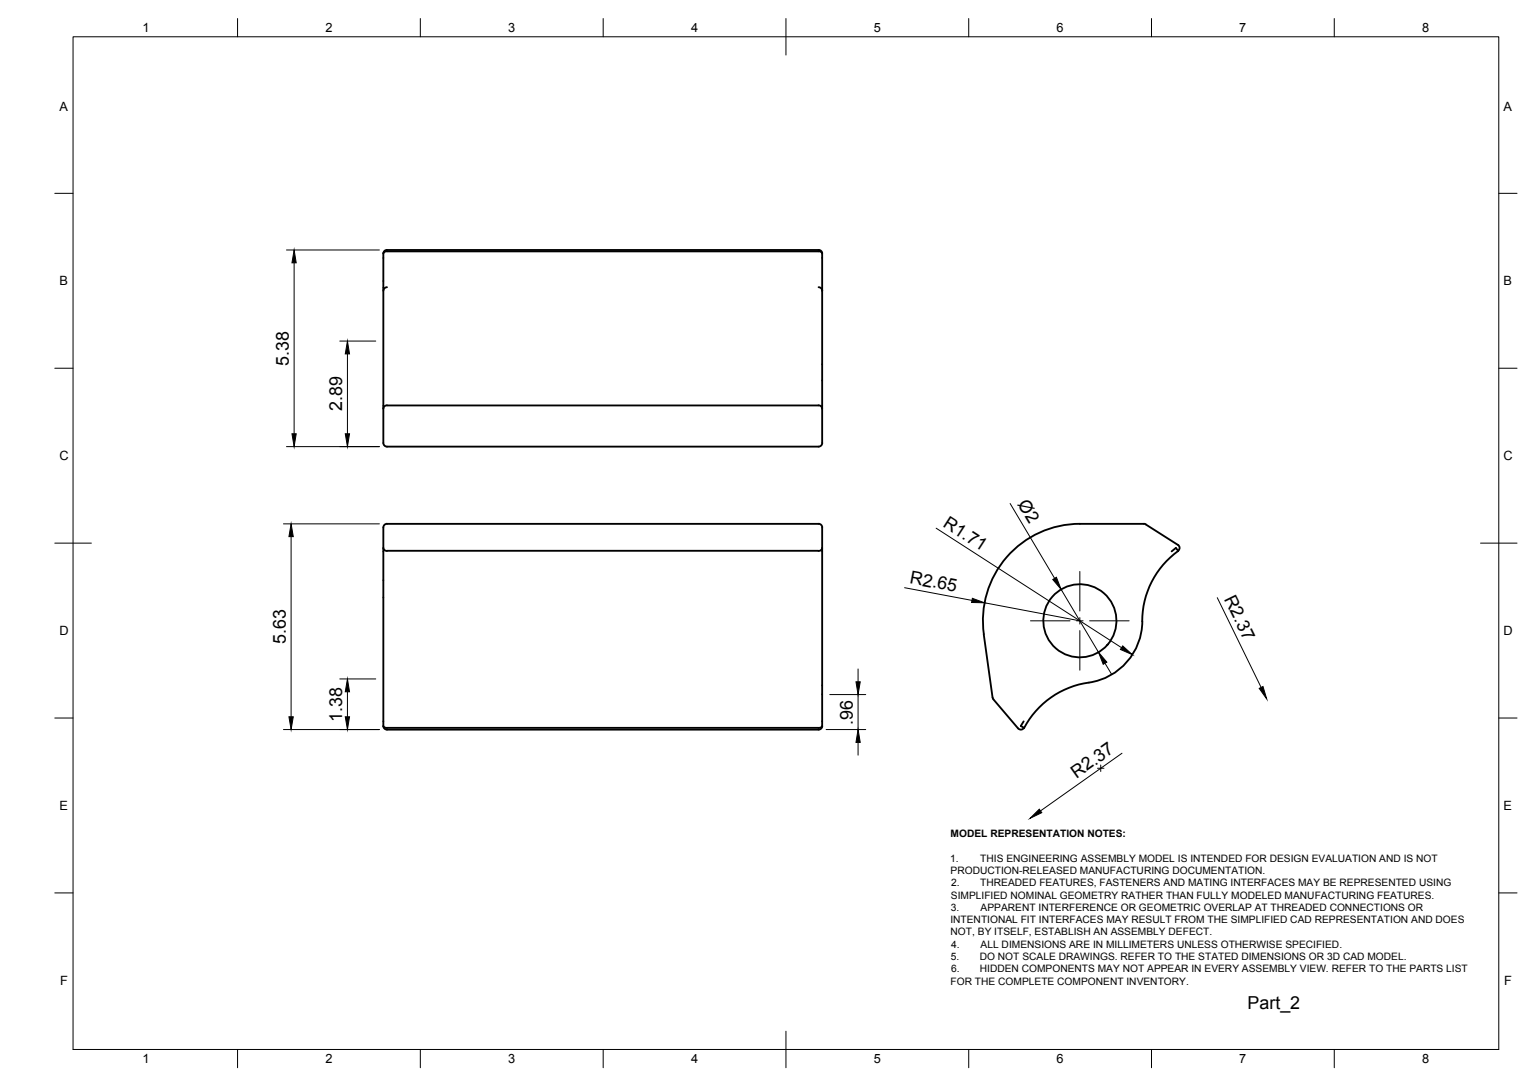
ISO-10303-21;
HEADER;
/* Generated by software containing ST-Developer
 * from STEP Tools, Inc. (www.steptools.com) 
 */

FILE_DESCRIPTION(
/* description */ ('STEP AP242 Edition 2'),
/* implementation_level */ '2;1');

FILE_NAME(
/* name */ 'Part_2.step',
/* time_stamp */ '2026-10-06T10:11:12-07:00',
/* author */ (''),
/* organization */ (''),
/* preprocessor_version */ 'ST-DEVELOPER v20.2',
/* originating_system */ 'Autodesk Translation Framework v15.15.0.0',
/* authorisation */ '');

FILE_SCHEMA (('AUTOMOTIVE_DESIGN { 1 0 10303 214 3 1 1 }'));
ENDSEC;

DATA;
#10=MECHANICAL_DESIGN_GEOMETRIC_PRESENTATION_REPRESENTATION('',(#1798),#54580);
#120=ELLIPSE('',#19218,0.0715418505295819,0.0129149243677278);
#121=ELLIPSE('',#19219,0.0715418505295819,0.0129149243677278);
#122=ELLIPSE('',#19224,0.0715418505290961,0.0129149243676839);
#123=ELLIPSE('',#19225,0.0715418505290961,0.0129149243676839);
#152=SPHERICAL_SURFACE('',#19236,0.0001);
#153=SPHERICAL_SURFACE('',#19238,0.0001);
#154=SPHERICAL_SURFACE('',#19251,0.0001);
#155=SPHERICAL_SURFACE('',#19256,0.0001);
#156=SPHERICAL_SURFACE('',#19270,0.0001);
#157=SPHERICAL_SURFACE('',#19273,0.0001);
#158=SPHERICAL_SURFACE('',#19284,0.0001);
#159=SPHERICAL_SURFACE('',#19286,0.0001);
#273=TOROIDAL_SURFACE('',#19243,0.0024677376190381,9.99991913251056E-5);
#274=TOROIDAL_SURFACE('',#19252,0.00160789487802693,0.0001);
#275=TOROIDAL_SURFACE('',#19254,0.00255162305984738,0.0001);
#276=TOROIDAL_SURFACE('',#19258,0.00246775438595658,9.99991912004813E-5);
#277=TOROIDAL_SURFACE('',#19259,0.00246775438598435,9.99991912004831E-5);
#278=TOROIDAL_SURFACE('',#19268,0.00160789487802693,0.0001);
#279=TOROIDAL_SURFACE('',#19275,0.00255162305984738,0.0001);
#280=TOROIDAL_SURFACE('',#19277,0.00246773761894624,9.99991913251039E-5);
#281=TOROIDAL_SURFACE('',#19289,0.0011,0.0001);
#282=TOROIDAL_SURFACE('',#19291,0.0011,0.0001);
#1352=B_SPLINE_CURVE_WITH_KNOTS('',3,(#48950,#48951,#48952,#48953),
 .UNSPECIFIED.,.F.,.F.,(4,4),(2.77758216759816E-8,0.0598155593219101),
 .UNSPECIFIED.);
#1353=B_SPLINE_CURVE_WITH_KNOTS('',3,(#48955,#48956,#48957,#48958,#48959,
#48960,#48961,#48962,#48963,#48964),.UNSPECIFIED.,.F.,.F.,(4,3,3,4),(0.0598155593219101,
0.400094789280781,0.882156340214427,1.),.UNSPECIFIED.);
#1354=B_SPLINE_CURVE_WITH_KNOTS('',3,(#48989,#48990,#48991,#48992),
 .UNSPECIFIED.,.F.,.F.,(4,4),(2.77758270156303E-8,0.0598155595006793),
 .UNSPECIFIED.);
#1355=B_SPLINE_CURVE_WITH_KNOTS('',3,(#48994,#48995,#48996,#48997,#48998,
#48999,#49000,#49001,#49002,#49003),.UNSPECIFIED.,.F.,.F.,(4,3,3,4),(0.0598155595006793,
0.400094789276241,0.882156340205139,1.),.UNSPECIFIED.);
#1356=B_SPLINE_CURVE_WITH_KNOTS('',3,(#49031,#49032,#49033,#49034,#49035,
#49036,#49037),.UNSPECIFIED.,.F.,.F.,(4,3,4),(0.,0.811097963900528,0.999989357516093),
 .UNSPECIFIED.);
#1357=B_SPLINE_CURVE_WITH_KNOTS('',3,(#49045,#49046,#49047,#49048,#49049,
#49050,#49051),.UNSPECIFIED.,.F.,.F.,(4,3,4),(0.,0.851452914537907,0.999998335389822),
 .UNSPECIFIED.);
#1358=B_SPLINE_CURVE_WITH_KNOTS('',3,(#49060,#49061,#49062,#49063,#49064,
#49065,#49066),.UNSPECIFIED.,.F.,.F.,(4,3,4),(0.000148834785990088,0.811264189000227,
1.),.UNSPECIFIED.);
#1359=B_SPLINE_CURVE_WITH_KNOTS('',3,(#49074,#49075,#49076,#49077,#49078,
#49079,#49080),.UNSPECIFIED.,.F.,.F.,(4,3,4),(1.66717332357201E-6,0.851450337612495,
1.),.UNSPECIFIED.);
#1360=B_SPLINE_CURVE_WITH_KNOTS('',3,(#49082,#49083,#49084,#49085,#49086,
#49087,#49088),.UNSPECIFIED.,.F.,.F.,(4,3,4),(0.00014883478557751,0.81126418904293,
1.),.UNSPECIFIED.);
#1361=B_SPLINE_CURVE_WITH_KNOTS('',3,(#49109,#49110,#49111,#49112,#49113,
#49114,#49115),.UNSPECIFIED.,.F.,.F.,(4,3,4),(0.,0.811097963770035,0.999989357516),
 .UNSPECIFIED.);
#1754=SHAPE_REPRESENTATION_RELATIONSHIP('SRR','None',#54641,#1768);
#1768=ADVANCED_BREP_SHAPE_REPRESENTATION('',(#1812),#54577);
#1798=STYLED_ITEM('',(#54712),#1812);
#1812=MANIFOLD_SOLID_BREP('Body1',#17677);
#2311=LINE('',#48890,#2904);
#2312=LINE('',#48894,#2905);
#2313=LINE('',#48899,#2906);
#2314=LINE('',#48901,#2907);
#2315=LINE('',#48903,#2908);
#2316=LINE('',#48904,#2909);
#2317=LINE('',#48908,#2910);
#2318=LINE('',#48910,#2911);
#2319=LINE('',#48912,#2912);
#2320=LINE('',#48913,#2913);
#2321=LINE('',#48918,#2914);
#2322=LINE('',#48922,#2915);
#2323=LINE('',#48924,#2916);
#2324=LINE('',#48925,#2917);
#2325=LINE('',#48929,#2918);
#2326=LINE('',#48931,#2919);
#2327=LINE('',#48933,#2920);
#2328=LINE('',#48934,#2921);
#2329=LINE('',#48938,#2922);
#2330=LINE('',#48942,#2923);
#2331=LINE('',#48972,#2924);
#2332=LINE('',#48974,#2925);
#2333=LINE('',#48978,#2926);
#2334=LINE('',#48979,#2927);
#2335=LINE('',#48985,#2928);
#2336=LINE('',#48987,#2929);
#2337=LINE('',#49011,#2930);
#2338=LINE('',#49013,#2931);
#2339=LINE('',#49023,#2932);
#2904=VECTOR('',#22829,0.01);
#2905=VECTOR('',#22832,0.01);
#2906=VECTOR('',#22837,1.);
#2907=VECTOR('',#22838,1.);
#2908=VECTOR('',#22839,1.);
#2909=VECTOR('',#22840,1.);
#2910=VECTOR('',#22843,1.);
#2911=VECTOR('',#22844,1.);
#2912=VECTOR('',#22845,1.);
#2913=VECTOR('',#22846,1.);
#2914=VECTOR('',#22851,1.);
#2915=VECTOR('',#22856,1.);
#2916=VECTOR('',#22857,1.);
#2917=VECTOR('',#22858,1.);
#2918=VECTOR('',#22861,1.);
#2919=VECTOR('',#22862,1.);
#2920=VECTOR('',#22863,1.);
#2921=VECTOR('',#22864,1.);
#2922=VECTOR('',#22867,0.01);
#2923=VECTOR('',#22870,0.01);
#2924=VECTOR('',#22887,1.);
#2925=VECTOR('',#22888,1.);
#2926=VECTOR('',#22891,1.);
#2927=VECTOR('',#22892,1.);
#2928=VECTOR('',#22897,1.);
#2929=VECTOR('',#22898,1.);
#2930=VECTOR('',#22905,1.);
#2931=VECTOR('',#22906,1.);
#2932=VECTOR('',#22917,0.001);
#3408=CYLINDRICAL_SURFACE('',#19200,0.00240582032312608);
#3409=CYLINDRICAL_SURFACE('',#19205,0.00265162305984738);
#3410=CYLINDRICAL_SURFACE('',#19210,0.00240582032360216);
#3411=CYLINDRICAL_SURFACE('',#19213,0.00170789487802692);
#3412=CYLINDRICAL_SURFACE('',#19228,0.001);
#3413=CYLINDRICAL_SURFACE('',#19233,0.0001);
#3414=CYLINDRICAL_SURFACE('',#19241,0.0001);
#3415=CYLINDRICAL_SURFACE('',#19244,0.0001);
#3416=CYLINDRICAL_SURFACE('',#19246,0.0001);
#3417=CYLINDRICAL_SURFACE('',#19248,0.0001);
#3418=CYLINDRICAL_SURFACE('',#19260,0.0001);
#3419=CYLINDRICAL_SURFACE('',#19264,0.0001);
#3420=CYLINDRICAL_SURFACE('',#19266,0.0001);
#3421=CYLINDRICAL_SURFACE('',#19278,0.0001);
#3422=CYLINDRICAL_SURFACE('',#19280,0.0001);
#3423=CYLINDRICAL_SURFACE('',#19282,0.0001);
#3424=CYLINDRICAL_SURFACE('',#19288,0.0001);
#3522=FACE_BOUND('',#5409,.T.);
#3523=FACE_BOUND('',#5411,.T.);
#4349=FACE_OUTER_BOUND('',#5400,.T.);
#4350=FACE_OUTER_BOUND('',#5401,.T.);
#4351=FACE_OUTER_BOUND('',#5402,.T.);
#4352=FACE_OUTER_BOUND('',#5403,.T.);
#4353=FACE_OUTER_BOUND('',#5404,.T.);
#4354=FACE_OUTER_BOUND('',#5405,.T.);
#4355=FACE_OUTER_BOUND('',#5406,.T.);
#4356=FACE_OUTER_BOUND('',#5407,.T.);
#4357=FACE_OUTER_BOUND('',#5408,.T.);
#4358=FACE_OUTER_BOUND('',#5410,.T.);
#4359=FACE_OUTER_BOUND('',#5412,.T.);
#4360=FACE_OUTER_BOUND('',#5413,.T.);
#4361=FACE_OUTER_BOUND('',#5414,.T.);
#4362=FACE_OUTER_BOUND('',#5415,.T.);
#4363=FACE_OUTER_BOUND('',#5416,.T.);
#4364=FACE_OUTER_BOUND('',#5417,.T.);
#4365=FACE_OUTER_BOUND('',#5418,.T.);
#4366=FACE_OUTER_BOUND('',#5419,.T.);
#4367=FACE_OUTER_BOUND('',#5420,.T.);
#4368=FACE_OUTER_BOUND('',#5421,.T.);
#4369=FACE_OUTER_BOUND('',#5422,.T.);
#4370=FACE_OUTER_BOUND('',#5423,.T.);
#4371=FACE_OUTER_BOUND('',#5424,.T.);
#4372=FACE_OUTER_BOUND('',#5425,.T.);
#4373=FACE_OUTER_BOUND('',#5426,.T.);
#4374=FACE_OUTER_BOUND('',#5427,.T.);
#4375=FACE_OUTER_BOUND('',#5428,.T.);
#4376=FACE_OUTER_BOUND('',#5429,.T.);
#4377=FACE_OUTER_BOUND('',#5430,.T.);
#4378=FACE_OUTER_BOUND('',#5431,.T.);
#4379=FACE_OUTER_BOUND('',#5432,.T.);
#4380=FACE_OUTER_BOUND('',#5433,.T.);
#4381=FACE_OUTER_BOUND('',#5434,.T.);
#4382=FACE_OUTER_BOUND('',#5435,.T.);
#4383=FACE_OUTER_BOUND('',#5436,.T.);
#4384=FACE_OUTER_BOUND('',#5437,.T.);
#4385=FACE_OUTER_BOUND('',#5438,.T.);
#4386=FACE_OUTER_BOUND('',#5439,.T.);
#4387=FACE_OUTER_BOUND('',#5440,.T.);
#4388=FACE_OUTER_BOUND('',#5441,.T.);
#4389=FACE_OUTER_BOUND('',#5442,.T.);
#5400=EDGE_LOOP('',(#15571,#15572,#15573,#15574));
#5401=EDGE_LOOP('',(#15575,#15576,#15577,#15578));
#5402=EDGE_LOOP('',(#15579,#15580,#15581,#15582));
#5403=EDGE_LOOP('',(#15583,#15584,#15585,#15586));
#5404=EDGE_LOOP('',(#15587,#15588,#15589,#15590));
#5405=EDGE_LOOP('',(#15591,#15592,#15593,#15594));
#5406=EDGE_LOOP('',(#15595,#15596,#15597,#15598));
#5407=EDGE_LOOP('',(#15599,#15600,#15601,#15602));
#5408=EDGE_LOOP('',(#15603,#15604,#15605,#15606,#15607,#15608,#15609,#15610,
#15611,#15612));
#5409=EDGE_LOOP('',(#15613));
#5410=EDGE_LOOP('',(#15614,#15615,#15616,#15617,#15618,#15619,#15620,#15621,
#15622,#15623));
#5411=EDGE_LOOP('',(#15624));
#5412=EDGE_LOOP('',(#15625,#15626,#15627,#15628,#15629,#15630));
#5413=EDGE_LOOP('',(#15631,#15632,#15633,#15634));
#5414=EDGE_LOOP('',(#15635,#15636,#15637));
#5415=EDGE_LOOP('',(#15638,#15639,#15640));
#5416=EDGE_LOOP('',(#15641,#15642,#15643,#15644));
#5417=EDGE_LOOP('',(#15645,#15646,#15647,#15648,#15649));
#5418=EDGE_LOOP('',(#15650,#15651,#15652,#15653));
#5419=EDGE_LOOP('',(#15654,#15655,#15656,#15657));
#5420=EDGE_LOOP('',(#15658,#15659,#15660,#15661));
#5421=EDGE_LOOP('',(#15662,#15663,#15664));
#5422=EDGE_LOOP('',(#15665,#15666,#15667,#15668));
#5423=EDGE_LOOP('',(#15669,#15670,#15671,#15672));
#5424=EDGE_LOOP('',(#15673,#15674,#15675));
#5425=EDGE_LOOP('',(#15676,#15677,#15678,#15679,#15680));
#5426=EDGE_LOOP('',(#15681,#15682,#15683,#15684,#15685));
#5427=EDGE_LOOP('',(#15686,#15687,#15688,#15689,#15690));
#5428=EDGE_LOOP('',(#15691,#15692,#15693,#15694));
#5429=EDGE_LOOP('',(#15695,#15696,#15697,#15698));
#5430=EDGE_LOOP('',(#15699,#15700,#15701,#15702));
#5431=EDGE_LOOP('',(#15703,#15704,#15705,#15706,#15707,#15708));
#5432=EDGE_LOOP('',(#15709,#15710,#15711));
#5433=EDGE_LOOP('',(#15712,#15713,#15714,#15715));
#5434=EDGE_LOOP('',(#15716,#15717,#15718,#15719,#15720));
#5435=EDGE_LOOP('',(#15721,#15722,#15723,#15724));
#5436=EDGE_LOOP('',(#15725,#15726,#15727,#15728));
#5437=EDGE_LOOP('',(#15729,#15730,#15731,#15732));
#5438=EDGE_LOOP('',(#15733,#15734,#15735));
#5439=EDGE_LOOP('',(#15736,#15737,#15738));
#5440=EDGE_LOOP('',(#15739,#15740,#15741,#15742));
#5441=EDGE_LOOP('',(#15743,#15744,#15745,#15746,#15747));
#5442=EDGE_LOOP('',(#15748,#15749,#15750,#15751,#15752));
#6312=CIRCLE('',#19201,0.00236773842762747);
#6313=CIRCLE('',#19202,0.00236775519479021);
#6314=CIRCLE('',#19206,0.00265162305984738);
#6315=CIRCLE('',#19207,0.00265162305984738);
#6316=CIRCLE('',#19211,0.00236775519476243);
#6317=CIRCLE('',#19212,0.00236773842771933);
#6318=CIRCLE('',#19214,0.00170789487802692);
#6319=CIRCLE('',#19215,0.00170789487802692);
#6320=CIRCLE('',#19217,0.00160789487802693);
#6321=CIRCLE('',#19220,0.00255162305984738);
#6322=CIRCLE('',#19221,0.0011);
#6323=CIRCLE('',#19223,0.00160789487802693);
#6324=CIRCLE('',#19226,0.00255162305984738);
#6325=CIRCLE('',#19227,0.0011);
#6326=CIRCLE('',#19229,0.001);
#6327=CIRCLE('',#19230,0.001);
#6328=CIRCLE('',#19231,0.001);
#6329=CIRCLE('',#19232,0.001);
#6330=CIRCLE('',#19234,0.0001);
#6331=CIRCLE('',#19235,0.0001);
#6332=CIRCLE('',#19237,0.0001);
#6333=CIRCLE('',#19239,0.0001);
#6334=CIRCLE('',#19240,0.0001);
#6335=CIRCLE('',#19242,0.0001);
#6336=CIRCLE('',#19245,0.0001);
#6337=CIRCLE('',#19247,0.0001);
#6338=CIRCLE('',#19249,0.0001);
#6339=CIRCLE('',#19250,0.0001);
#6340=CIRCLE('',#19253,0.000100001088290115);
#6341=CIRCLE('',#19255,0.0001);
#6342=CIRCLE('',#19257,0.0001);
#6343=CIRCLE('',#19261,0.0001);
#6344=CIRCLE('',#19262,0.0001);
#6345=CIRCLE('',#19263,0.0001);
#6346=CIRCLE('',#19265,0.0001);
#6347=CIRCLE('',#19267,0.0001);
#6348=CIRCLE('',#19269,0.000100001089498111);
#6349=CIRCLE('',#19271,9.99999999999998E-5);
#6350=CIRCLE('',#19272,0.0001);
#6351=CIRCLE('',#19274,0.0001);
#6352=CIRCLE('',#19276,0.0001);
#6353=CIRCLE('',#19279,0.0001);
#6354=CIRCLE('',#19281,0.0001);
#6355=CIRCLE('',#19283,0.0001);
#6356=CIRCLE('',#19285,0.0001);
#6357=CIRCLE('',#19287,0.0001);
#6358=CIRCLE('',#19290,0.0001);
#6359=CIRCLE('',#19292,0.0001);
#8021=VERTEX_POINT('',#48888);
#8022=VERTEX_POINT('',#48889);
#8023=VERTEX_POINT('',#48891);
#8024=VERTEX_POINT('',#48893);
#8025=VERTEX_POINT('',#48897);
#8026=VERTEX_POINT('',#48898);
#8027=VERTEX_POINT('',#48900);
#8028=VERTEX_POINT('',#48902);
#8029=VERTEX_POINT('',#48906);
#8030=VERTEX_POINT('',#48907);
#8031=VERTEX_POINT('',#48909);
#8032=VERTEX_POINT('',#48911);
#8033=VERTEX_POINT('',#48915);
#8034=VERTEX_POINT('',#48917);
#8035=VERTEX_POINT('',#48921);
#8036=VERTEX_POINT('',#48923);
#8037=VERTEX_POINT('',#48927);
#8038=VERTEX_POINT('',#48928);
#8039=VERTEX_POINT('',#48930);
#8040=VERTEX_POINT('',#48932);
#8041=VERTEX_POINT('',#48936);
#8042=VERTEX_POINT('',#48937);
#8043=VERTEX_POINT('',#48939);
#8044=VERTEX_POINT('',#48941);
#8045=VERTEX_POINT('',#48948);
#8046=VERTEX_POINT('',#48949);
#8047=VERTEX_POINT('',#48954);
#8048=VERTEX_POINT('',#48965);
#8049=VERTEX_POINT('',#48967);
#8050=VERTEX_POINT('',#48969);
#8051=VERTEX_POINT('',#48971);
#8052=VERTEX_POINT('',#48973);
#8053=VERTEX_POINT('',#48975);
#8054=VERTEX_POINT('',#48977);
#8055=VERTEX_POINT('',#48980);
#8056=VERTEX_POINT('',#48983);
#8057=VERTEX_POINT('',#48984);
#8058=VERTEX_POINT('',#48986);
#8059=VERTEX_POINT('',#48988);
#8060=VERTEX_POINT('',#48993);
#8061=VERTEX_POINT('',#49004);
#8062=VERTEX_POINT('',#49006);
#8063=VERTEX_POINT('',#49008);
#8064=VERTEX_POINT('',#49010);
#8065=VERTEX_POINT('',#49012);
#8066=VERTEX_POINT('',#49015);
#8067=VERTEX_POINT('',#49018);
#8068=VERTEX_POINT('',#49019);
#8069=VERTEX_POINT('',#49022);
#8070=VERTEX_POINT('',#49024);
#8071=VERTEX_POINT('',#49091);
#8072=VERTEX_POINT('',#49101);
#10577=EDGE_CURVE('',#8021,#8022,#2311,.T.);
#10578=EDGE_CURVE('',#8022,#8023,#6312,.T.);
#10579=EDGE_CURVE('',#8023,#8024,#2312,.T.);
#10580=EDGE_CURVE('',#8024,#8021,#6313,.T.);
#10581=EDGE_CURVE('',#8025,#8026,#2313,.T.);
#10582=EDGE_CURVE('',#8026,#8027,#2314,.F.);
#10583=EDGE_CURVE('',#8027,#8028,#2315,.F.);
#10584=EDGE_CURVE('',#8028,#8025,#2316,.T.);
#10585=EDGE_CURVE('',#8029,#8030,#2317,.T.);
#10586=EDGE_CURVE('',#8030,#8031,#2318,.T.);
#10587=EDGE_CURVE('',#8032,#8031,#2319,.T.);
#10588=EDGE_CURVE('',#8032,#8029,#2320,.F.);
#10589=EDGE_CURVE('',#8031,#8033,#6314,.F.);
#10590=EDGE_CURVE('',#8034,#8033,#2321,.T.);
#10591=EDGE_CURVE('',#8034,#8032,#6315,.T.);
#10592=EDGE_CURVE('',#8033,#8035,#2322,.T.);
#10593=EDGE_CURVE('',#8035,#8036,#2323,.F.);
#10594=EDGE_CURVE('',#8036,#8034,#2324,.F.);
#10595=EDGE_CURVE('',#8037,#8038,#2325,.F.);
#10596=EDGE_CURVE('',#8038,#8039,#2326,.T.);
#10597=EDGE_CURVE('',#8039,#8040,#2327,.T.);
#10598=EDGE_CURVE('',#8040,#8037,#2328,.F.);
#10599=EDGE_CURVE('',#8041,#8042,#2329,.T.);
#10600=EDGE_CURVE('',#8042,#8043,#6316,.T.);
#10601=EDGE_CURVE('',#8044,#8043,#2330,.F.);
#10602=EDGE_CURVE('',#8044,#8041,#6317,.T.);
#10603=EDGE_CURVE('',#8043,#8022,#6318,.F.);
#10604=EDGE_CURVE('',#8021,#8044,#6319,.T.);
#10605=EDGE_CURVE('',#8045,#8046,#1352,.T.);
#10606=EDGE_CURVE('',#8046,#8047,#1353,.T.);
#10607=EDGE_CURVE('',#8047,#8048,#6320,.F.);
#10608=EDGE_CURVE('',#8048,#8049,#120,.T.);
#10609=EDGE_CURVE('',#8049,#8050,#121,.T.);
#10610=EDGE_CURVE('',#8050,#8051,#2331,.T.);
#10611=EDGE_CURVE('',#8051,#8052,#2332,.T.);
#10612=EDGE_CURVE('',#8052,#8053,#6321,.F.);
#10613=EDGE_CURVE('',#8053,#8054,#2333,.T.);
#10614=EDGE_CURVE('',#8054,#8045,#2334,.T.);
#10615=EDGE_CURVE('',#8055,#8055,#6322,.T.);
#10616=EDGE_CURVE('',#8056,#8057,#2335,.F.);
#10617=EDGE_CURVE('',#8057,#8058,#2336,.F.);
#10618=EDGE_CURVE('',#8058,#8059,#1354,.T.);
#10619=EDGE_CURVE('',#8059,#8060,#1355,.T.);
#10620=EDGE_CURVE('',#8060,#8061,#6323,.T.);
#10621=EDGE_CURVE('',#8061,#8062,#122,.T.);
#10622=EDGE_CURVE('',#8062,#8063,#123,.T.);
#10623=EDGE_CURVE('',#8063,#8064,#2337,.F.);
#10624=EDGE_CURVE('',#8064,#8065,#2338,.F.);
#10625=EDGE_CURVE('',#8065,#8056,#6324,.T.);
#10626=EDGE_CURVE('',#8066,#8066,#6325,.F.);
#10627=EDGE_CURVE('',#8067,#8068,#6326,.T.);
#10628=EDGE_CURVE('',#8068,#8067,#6327,.T.);
#10629=EDGE_CURVE('',#8067,#8069,#2339,.T.);
#10630=EDGE_CURVE('',#8069,#8070,#6328,.F.);
#10631=EDGE_CURVE('',#8070,#8069,#6329,.F.);
#10632=EDGE_CURVE('',#8045,#8037,#6330,.T.);
#10633=EDGE_CURVE('',#8038,#8054,#6331,.T.);
#10634=EDGE_CURVE('',#8045,#8041,#1356,.F.);
#10635=EDGE_CURVE('',#8041,#8037,#6332,.F.);
#10636=EDGE_CURVE('',#8038,#8036,#6333,.F.);
#10637=EDGE_CURVE('',#8036,#8054,#6334,.F.);
#10638=EDGE_CURVE('',#8042,#8040,#6335,.T.);
#10639=EDGE_CURVE('',#8047,#8044,#1357,.F.);
#10640=EDGE_CURVE('',#8034,#8053,#6336,.T.);
#10641=EDGE_CURVE('',#8039,#8035,#6337,.T.);
#10642=EDGE_CURVE('',#8040,#8063,#6338,.T.);
#10643=EDGE_CURVE('',#8064,#8039,#6339,.T.);
#10644=EDGE_CURVE('',#8042,#8063,#1358,.F.);
#10645=EDGE_CURVE('',#8048,#8021,#6340,.F.);
#10646=EDGE_CURVE('',#8032,#8052,#6341,.T.);
#10647=EDGE_CURVE('',#8064,#8035,#6342,.F.);
#10648=EDGE_CURVE('',#8043,#8061,#1359,.F.);
#10649=EDGE_CURVE('',#8050,#8024,#1360,.T.);
#10650=EDGE_CURVE('',#8051,#8027,#6343,.T.);
#10651=EDGE_CURVE('',#8071,#8050,#6344,.T.);
#10652=EDGE_CURVE('',#8028,#8071,#6345,.T.);
#10653=EDGE_CURVE('',#8029,#8051,#6346,.T.);
#10654=EDGE_CURVE('',#8065,#8033,#6347,.T.);
#10655=EDGE_CURVE('',#8022,#8060,#6348,.F.);
#10656=EDGE_CURVE('',#8072,#8071,#6349,.T.);
#10657=EDGE_CURVE('',#8028,#8024,#6350,.F.);
#10658=EDGE_CURVE('',#8029,#8027,#6351,.F.);
#10659=EDGE_CURVE('',#8056,#8031,#6352,.T.);
#10660=EDGE_CURVE('',#8023,#8058,#1361,.T.);
#10661=EDGE_CURVE('',#8025,#8023,#6353,.T.);
#10662=EDGE_CURVE('',#8030,#8026,#6354,.T.);
#10663=EDGE_CURVE('',#8057,#8030,#6355,.T.);
#10664=EDGE_CURVE('',#8025,#8058,#6356,.F.);
#10665=EDGE_CURVE('',#8057,#8026,#6357,.F.);
#10666=EDGE_CURVE('',#8068,#8066,#6358,.T.);
#10667=EDGE_CURVE('',#8055,#8070,#6359,.T.);
#15571=ORIENTED_EDGE('',*,*,#10577,.T.);
#15572=ORIENTED_EDGE('',*,*,#10578,.T.);
#15573=ORIENTED_EDGE('',*,*,#10579,.T.);
#15574=ORIENTED_EDGE('',*,*,#10580,.T.);
#15575=ORIENTED_EDGE('',*,*,#10581,.T.);
#15576=ORIENTED_EDGE('',*,*,#10582,.T.);
#15577=ORIENTED_EDGE('',*,*,#10583,.T.);
#15578=ORIENTED_EDGE('',*,*,#10584,.T.);
#15579=ORIENTED_EDGE('',*,*,#10585,.T.);
#15580=ORIENTED_EDGE('',*,*,#10586,.T.);
#15581=ORIENTED_EDGE('',*,*,#10587,.F.);
#15582=ORIENTED_EDGE('',*,*,#10588,.T.);
#15583=ORIENTED_EDGE('',*,*,#10587,.T.);
#15584=ORIENTED_EDGE('',*,*,#10589,.T.);
#15585=ORIENTED_EDGE('',*,*,#10590,.F.);
#15586=ORIENTED_EDGE('',*,*,#10591,.T.);
#15587=ORIENTED_EDGE('',*,*,#10590,.T.);
#15588=ORIENTED_EDGE('',*,*,#10592,.T.);
#15589=ORIENTED_EDGE('',*,*,#10593,.T.);
#15590=ORIENTED_EDGE('',*,*,#10594,.T.);
#15591=ORIENTED_EDGE('',*,*,#10595,.T.);
#15592=ORIENTED_EDGE('',*,*,#10596,.T.);
#15593=ORIENTED_EDGE('',*,*,#10597,.T.);
#15594=ORIENTED_EDGE('',*,*,#10598,.T.);
#15595=ORIENTED_EDGE('',*,*,#10599,.T.);
#15596=ORIENTED_EDGE('',*,*,#10600,.T.);
#15597=ORIENTED_EDGE('',*,*,#10601,.F.);
#15598=ORIENTED_EDGE('',*,*,#10602,.T.);
#15599=ORIENTED_EDGE('',*,*,#10601,.T.);
#15600=ORIENTED_EDGE('',*,*,#10603,.T.);
#15601=ORIENTED_EDGE('',*,*,#10577,.F.);
#15602=ORIENTED_EDGE('',*,*,#10604,.T.);
#15603=ORIENTED_EDGE('',*,*,#10605,.T.);
#15604=ORIENTED_EDGE('',*,*,#10606,.T.);
#15605=ORIENTED_EDGE('',*,*,#10607,.T.);
#15606=ORIENTED_EDGE('',*,*,#10608,.T.);
#15607=ORIENTED_EDGE('',*,*,#10609,.T.);
#15608=ORIENTED_EDGE('',*,*,#10610,.T.);
#15609=ORIENTED_EDGE('',*,*,#10611,.T.);
#15610=ORIENTED_EDGE('',*,*,#10612,.T.);
#15611=ORIENTED_EDGE('',*,*,#10613,.T.);
#15612=ORIENTED_EDGE('',*,*,#10614,.T.);
#15613=ORIENTED_EDGE('',*,*,#10615,.T.);
#15614=ORIENTED_EDGE('',*,*,#10616,.T.);
#15615=ORIENTED_EDGE('',*,*,#10617,.T.);
#15616=ORIENTED_EDGE('',*,*,#10618,.T.);
#15617=ORIENTED_EDGE('',*,*,#10619,.T.);
#15618=ORIENTED_EDGE('',*,*,#10620,.T.);
#15619=ORIENTED_EDGE('',*,*,#10621,.T.);
#15620=ORIENTED_EDGE('',*,*,#10622,.T.);
#15621=ORIENTED_EDGE('',*,*,#10623,.T.);
#15622=ORIENTED_EDGE('',*,*,#10624,.T.);
#15623=ORIENTED_EDGE('',*,*,#10625,.T.);
#15624=ORIENTED_EDGE('',*,*,#10626,.T.);
#15625=ORIENTED_EDGE('',*,*,#10627,.T.);
#15626=ORIENTED_EDGE('',*,*,#10628,.T.);
#15627=ORIENTED_EDGE('',*,*,#10629,.T.);
#15628=ORIENTED_EDGE('',*,*,#10630,.T.);
#15629=ORIENTED_EDGE('',*,*,#10631,.T.);
#15630=ORIENTED_EDGE('',*,*,#10629,.F.);
#15631=ORIENTED_EDGE('',*,*,#10632,.F.);
#15632=ORIENTED_EDGE('',*,*,#10614,.F.);
#15633=ORIENTED_EDGE('',*,*,#10633,.F.);
#15634=ORIENTED_EDGE('',*,*,#10595,.F.);
#15635=ORIENTED_EDGE('',*,*,#10634,.F.);
#15636=ORIENTED_EDGE('',*,*,#10632,.T.);
#15637=ORIENTED_EDGE('',*,*,#10635,.F.);
#15638=ORIENTED_EDGE('',*,*,#10636,.F.);
#15639=ORIENTED_EDGE('',*,*,#10633,.T.);
#15640=ORIENTED_EDGE('',*,*,#10637,.F.);
#15641=ORIENTED_EDGE('',*,*,#10635,.T.);
#15642=ORIENTED_EDGE('',*,*,#10598,.F.);
#15643=ORIENTED_EDGE('',*,*,#10638,.F.);
#15644=ORIENTED_EDGE('',*,*,#10599,.F.);
#15645=ORIENTED_EDGE('',*,*,#10634,.T.);
#15646=ORIENTED_EDGE('',*,*,#10602,.F.);
#15647=ORIENTED_EDGE('',*,*,#10639,.F.);
#15648=ORIENTED_EDGE('',*,*,#10606,.F.);
#15649=ORIENTED_EDGE('',*,*,#10605,.F.);
#15650=ORIENTED_EDGE('',*,*,#10637,.T.);
#15651=ORIENTED_EDGE('',*,*,#10613,.F.);
#15652=ORIENTED_EDGE('',*,*,#10640,.F.);
#15653=ORIENTED_EDGE('',*,*,#10594,.F.);
#15654=ORIENTED_EDGE('',*,*,#10636,.T.);
#15655=ORIENTED_EDGE('',*,*,#10593,.F.);
#15656=ORIENTED_EDGE('',*,*,#10641,.F.);
#15657=ORIENTED_EDGE('',*,*,#10596,.F.);
#15658=ORIENTED_EDGE('',*,*,#10642,.F.);
#15659=ORIENTED_EDGE('',*,*,#10597,.F.);
#15660=ORIENTED_EDGE('',*,*,#10643,.F.);
#15661=ORIENTED_EDGE('',*,*,#10623,.F.);
#15662=ORIENTED_EDGE('',*,*,#10638,.T.);
#15663=ORIENTED_EDGE('',*,*,#10642,.T.);
#15664=ORIENTED_EDGE('',*,*,#10644,.F.);
#15665=ORIENTED_EDGE('',*,*,#10639,.T.);
#15666=ORIENTED_EDGE('',*,*,#10604,.F.);
#15667=ORIENTED_EDGE('',*,*,#10645,.F.);
#15668=ORIENTED_EDGE('',*,*,#10607,.F.);
#15669=ORIENTED_EDGE('',*,*,#10640,.T.);
#15670=ORIENTED_EDGE('',*,*,#10612,.F.);
#15671=ORIENTED_EDGE('',*,*,#10646,.F.);
#15672=ORIENTED_EDGE('',*,*,#10591,.F.);
#15673=ORIENTED_EDGE('',*,*,#10643,.T.);
#15674=ORIENTED_EDGE('',*,*,#10641,.T.);
#15675=ORIENTED_EDGE('',*,*,#10647,.F.);
#15676=ORIENTED_EDGE('',*,*,#10644,.T.);
#15677=ORIENTED_EDGE('',*,*,#10622,.F.);
#15678=ORIENTED_EDGE('',*,*,#10621,.F.);
#15679=ORIENTED_EDGE('',*,*,#10648,.F.);
#15680=ORIENTED_EDGE('',*,*,#10600,.F.);
#15681=ORIENTED_EDGE('',*,*,#10645,.T.);
#15682=ORIENTED_EDGE('',*,*,#10580,.F.);
#15683=ORIENTED_EDGE('',*,*,#10649,.F.);
#15684=ORIENTED_EDGE('',*,*,#10609,.F.);
#15685=ORIENTED_EDGE('',*,*,#10608,.F.);
#15686=ORIENTED_EDGE('',*,*,#10650,.F.);
#15687=ORIENTED_EDGE('',*,*,#10610,.F.);
#15688=ORIENTED_EDGE('',*,*,#10651,.F.);
#15689=ORIENTED_EDGE('',*,*,#10652,.F.);
#15690=ORIENTED_EDGE('',*,*,#10583,.F.);
#15691=ORIENTED_EDGE('',*,*,#10646,.T.);
#15692=ORIENTED_EDGE('',*,*,#10611,.F.);
#15693=ORIENTED_EDGE('',*,*,#10653,.F.);
#15694=ORIENTED_EDGE('',*,*,#10588,.F.);
#15695=ORIENTED_EDGE('',*,*,#10647,.T.);
#15696=ORIENTED_EDGE('',*,*,#10592,.F.);
#15697=ORIENTED_EDGE('',*,*,#10654,.F.);
#15698=ORIENTED_EDGE('',*,*,#10624,.F.);
#15699=ORIENTED_EDGE('',*,*,#10648,.T.);
#15700=ORIENTED_EDGE('',*,*,#10620,.F.);
#15701=ORIENTED_EDGE('',*,*,#10655,.F.);
#15702=ORIENTED_EDGE('',*,*,#10603,.F.);
#15703=ORIENTED_EDGE('',*,*,#10652,.T.);
#15704=ORIENTED_EDGE('',*,*,#10656,.F.);
#15705=ORIENTED_EDGE('',*,*,#10656,.T.);
#15706=ORIENTED_EDGE('',*,*,#10651,.T.);
#15707=ORIENTED_EDGE('',*,*,#10649,.T.);
#15708=ORIENTED_EDGE('',*,*,#10657,.F.);
#15709=ORIENTED_EDGE('',*,*,#10653,.T.);
#15710=ORIENTED_EDGE('',*,*,#10650,.T.);
#15711=ORIENTED_EDGE('',*,*,#10658,.F.);
#15712=ORIENTED_EDGE('',*,*,#10654,.T.);
#15713=ORIENTED_EDGE('',*,*,#10589,.F.);
#15714=ORIENTED_EDGE('',*,*,#10659,.F.);
#15715=ORIENTED_EDGE('',*,*,#10625,.F.);
#15716=ORIENTED_EDGE('',*,*,#10655,.T.);
#15717=ORIENTED_EDGE('',*,*,#10619,.F.);
#15718=ORIENTED_EDGE('',*,*,#10618,.F.);
#15719=ORIENTED_EDGE('',*,*,#10660,.F.);
#15720=ORIENTED_EDGE('',*,*,#10578,.F.);
#15721=ORIENTED_EDGE('',*,*,#10657,.T.);
#15722=ORIENTED_EDGE('',*,*,#10579,.F.);
#15723=ORIENTED_EDGE('',*,*,#10661,.F.);
#15724=ORIENTED_EDGE('',*,*,#10584,.F.);
#15725=ORIENTED_EDGE('',*,*,#10658,.T.);
#15726=ORIENTED_EDGE('',*,*,#10582,.F.);
#15727=ORIENTED_EDGE('',*,*,#10662,.F.);
#15728=ORIENTED_EDGE('',*,*,#10585,.F.);
#15729=ORIENTED_EDGE('',*,*,#10659,.T.);
#15730=ORIENTED_EDGE('',*,*,#10586,.F.);
#15731=ORIENTED_EDGE('',*,*,#10663,.F.);
#15732=ORIENTED_EDGE('',*,*,#10616,.F.);
#15733=ORIENTED_EDGE('',*,*,#10661,.T.);
#15734=ORIENTED_EDGE('',*,*,#10660,.T.);
#15735=ORIENTED_EDGE('',*,*,#10664,.F.);
#15736=ORIENTED_EDGE('',*,*,#10663,.T.);
#15737=ORIENTED_EDGE('',*,*,#10662,.T.);
#15738=ORIENTED_EDGE('',*,*,#10665,.F.);
#15739=ORIENTED_EDGE('',*,*,#10664,.T.);
#15740=ORIENTED_EDGE('',*,*,#10617,.F.);
#15741=ORIENTED_EDGE('',*,*,#10665,.T.);
#15742=ORIENTED_EDGE('',*,*,#10581,.F.);
#15743=ORIENTED_EDGE('',*,*,#10627,.F.);
#15744=ORIENTED_EDGE('',*,*,#10628,.F.);
#15745=ORIENTED_EDGE('',*,*,#10666,.T.);
#15746=ORIENTED_EDGE('',*,*,#10626,.F.);
#15747=ORIENTED_EDGE('',*,*,#10666,.F.);
#15748=ORIENTED_EDGE('',*,*,#10615,.F.);
#15749=ORIENTED_EDGE('',*,*,#10667,.T.);
#15750=ORIENTED_EDGE('',*,*,#10630,.F.);
#15751=ORIENTED_EDGE('',*,*,#10631,.F.);
#15752=ORIENTED_EDGE('',*,*,#10667,.F.);
#16639=PLANE('',#19203);
#16640=PLANE('',#19204);
#16641=PLANE('',#19208);
#16642=PLANE('',#19209);
#16643=PLANE('',#19216);
#16644=PLANE('',#19222);
#17465=ADVANCED_FACE('',(#4349),#3408,.F.);
#17466=ADVANCED_FACE('',(#4350),#16639,.F.);
#17467=ADVANCED_FACE('',(#4351),#16640,.F.);
#17468=ADVANCED_FACE('',(#4352),#3409,.T.);
#17469=ADVANCED_FACE('',(#4353),#16641,.F.);
#17470=ADVANCED_FACE('',(#4354),#16642,.F.);
#17471=ADVANCED_FACE('',(#4355),#3410,.F.);
#17472=ADVANCED_FACE('',(#4356),#3411,.T.);
#17473=ADVANCED_FACE('',(#4357,#3522),#16643,.F.);
#17474=ADVANCED_FACE('',(#4358,#3523),#16644,.T.);
#17475=ADVANCED_FACE('',(#4359),#3412,.F.);
#17476=ADVANCED_FACE('',(#4360),#3413,.T.);
#17477=ADVANCED_FACE('',(#4361),#152,.T.);
#17478=ADVANCED_FACE('',(#4362),#153,.T.);
#17479=ADVANCED_FACE('',(#4363),#3414,.T.);
#17480=ADVANCED_FACE('',(#4364),#273,.T.);
#17481=ADVANCED_FACE('',(#4365),#3415,.T.);
#17482=ADVANCED_FACE('',(#4366),#3416,.T.);
#17483=ADVANCED_FACE('',(#4367),#3417,.T.);
#17484=ADVANCED_FACE('',(#4368),#154,.T.);
#17485=ADVANCED_FACE('',(#4369),#274,.T.);
#17486=ADVANCED_FACE('',(#4370),#275,.T.);
#17487=ADVANCED_FACE('',(#4371),#155,.T.);
#17488=ADVANCED_FACE('',(#4372),#276,.T.);
#17489=ADVANCED_FACE('',(#4373),#277,.T.);
#17490=ADVANCED_FACE('',(#4374),#3418,.T.);
#17491=ADVANCED_FACE('',(#4375),#3419,.T.);
#17492=ADVANCED_FACE('',(#4376),#3420,.T.);
#17493=ADVANCED_FACE('',(#4377),#278,.T.);
#17494=ADVANCED_FACE('',(#4378),#156,.T.);
#17495=ADVANCED_FACE('',(#4379),#157,.T.);
#17496=ADVANCED_FACE('',(#4380),#279,.T.);
#17497=ADVANCED_FACE('',(#4381),#280,.T.);
#17498=ADVANCED_FACE('',(#4382),#3421,.T.);
#17499=ADVANCED_FACE('',(#4383),#3422,.T.);
#17500=ADVANCED_FACE('',(#4384),#3423,.T.);
#17501=ADVANCED_FACE('',(#4385),#158,.T.);
#17502=ADVANCED_FACE('',(#4386),#159,.T.);
#17503=ADVANCED_FACE('',(#4387),#3424,.T.);
#17504=ADVANCED_FACE('',(#4388),#281,.T.);
#17505=ADVANCED_FACE('',(#4389),#282,.T.);
#17677=CLOSED_SHELL('',(#17465,#17466,#17467,#17468,#17469,#17470,#17471,
#17472,#17473,#17474,#17475,#17476,#17477,#17478,#17479,#17480,#17481,#17482,
#17483,#17484,#17485,#17486,#17487,#17488,#17489,#17490,#17491,#17492,#17493,
#17494,#17495,#17496,#17497,#17498,#17499,#17500,#17501,#17502,#17503,#17504,
#17505));
#19199=AXIS2_PLACEMENT_3D('',#48886,#22825,#22826);
#19200=AXIS2_PLACEMENT_3D('',#48887,#22827,#22828);
#19201=AXIS2_PLACEMENT_3D('',#48892,#22830,#22831);
#19202=AXIS2_PLACEMENT_3D('',#48895,#22833,#22834);
#19203=AXIS2_PLACEMENT_3D('',#48896,#22835,#22836);
#19204=AXIS2_PLACEMENT_3D('',#48905,#22841,#22842);
#19205=AXIS2_PLACEMENT_3D('',#48914,#22847,#22848);
#19206=AXIS2_PLACEMENT_3D('',#48916,#22849,#22850);
#19207=AXIS2_PLACEMENT_3D('',#48919,#22852,#22853);
#19208=AXIS2_PLACEMENT_3D('',#48920,#22854,#22855);
#19209=AXIS2_PLACEMENT_3D('',#48926,#22859,#22860);
#19210=AXIS2_PLACEMENT_3D('',#48935,#22865,#22866);
#19211=AXIS2_PLACEMENT_3D('',#48940,#22868,#22869);
#19212=AXIS2_PLACEMENT_3D('',#48943,#22871,#22872);
#19213=AXIS2_PLACEMENT_3D('',#48944,#22873,#22874);
#19214=AXIS2_PLACEMENT_3D('',#48945,#22875,#22876);
#19215=AXIS2_PLACEMENT_3D('',#48946,#22877,#22878);
#19216=AXIS2_PLACEMENT_3D('',#48947,#22879,#22880);
#19217=AXIS2_PLACEMENT_3D('',#48966,#22881,#22882);
#19218=AXIS2_PLACEMENT_3D('',#48968,#22883,#22884);
#19219=AXIS2_PLACEMENT_3D('',#48970,#22885,#22886);
#19220=AXIS2_PLACEMENT_3D('',#48976,#22889,#22890);
#19221=AXIS2_PLACEMENT_3D('',#48981,#22893,#22894);
#19222=AXIS2_PLACEMENT_3D('',#48982,#22895,#22896);
#19223=AXIS2_PLACEMENT_3D('',#49005,#22899,#22900);
#19224=AXIS2_PLACEMENT_3D('',#49007,#22901,#22902);
#19225=AXIS2_PLACEMENT_3D('',#49009,#22903,#22904);
#19226=AXIS2_PLACEMENT_3D('',#49014,#22907,#22908);
#19227=AXIS2_PLACEMENT_3D('',#49016,#22909,#22910);
#19228=AXIS2_PLACEMENT_3D('',#49017,#22911,#22912);
#19229=AXIS2_PLACEMENT_3D('',#49020,#22913,#22914);
#19230=AXIS2_PLACEMENT_3D('',#49021,#22915,#22916);
#19231=AXIS2_PLACEMENT_3D('',#49025,#22918,#22919);
#19232=AXIS2_PLACEMENT_3D('',#49026,#22920,#22921);
#19233=AXIS2_PLACEMENT_3D('',#49027,#22922,#22923);
#19234=AXIS2_PLACEMENT_3D('',#49028,#22924,#22925);
#19235=AXIS2_PLACEMENT_3D('',#49029,#22926,#22927);
#19236=AXIS2_PLACEMENT_3D('',#49030,#22928,#22929);
#19237=AXIS2_PLACEMENT_3D('',#49038,#22930,#22931);
#19238=AXIS2_PLACEMENT_3D('',#49039,#22932,#22933);
#19239=AXIS2_PLACEMENT_3D('',#49040,#22934,#22935);
#19240=AXIS2_PLACEMENT_3D('',#49041,#22936,#22937);
#19241=AXIS2_PLACEMENT_3D('',#49042,#22938,#22939);
#19242=AXIS2_PLACEMENT_3D('',#49043,#22940,#22941);
#19243=AXIS2_PLACEMENT_3D('',#49044,#22942,#22943);
#19244=AXIS2_PLACEMENT_3D('',#49052,#22944,#22945);
#19245=AXIS2_PLACEMENT_3D('',#49053,#22946,#22947);
#19246=AXIS2_PLACEMENT_3D('',#49054,#22948,#22949);
#19247=AXIS2_PLACEMENT_3D('',#49055,#22950,#22951);
#19248=AXIS2_PLACEMENT_3D('',#49056,#22952,#22953);
#19249=AXIS2_PLACEMENT_3D('',#49057,#22954,#22955);
#19250=AXIS2_PLACEMENT_3D('',#49058,#22956,#22957);
#19251=AXIS2_PLACEMENT_3D('',#49059,#22958,#22959);
#19252=AXIS2_PLACEMENT_3D('',#49067,#22960,#22961);
#19253=AXIS2_PLACEMENT_3D('',#49068,#22962,#22963);
#19254=AXIS2_PLACEMENT_3D('',#49069,#22964,#22965);
#19255=AXIS2_PLACEMENT_3D('',#49070,#22966,#22967);
#19256=AXIS2_PLACEMENT_3D('',#49071,#22968,#22969);
#19257=AXIS2_PLACEMENT_3D('',#49072,#22970,#22971);
#19258=AXIS2_PLACEMENT_3D('',#49073,#22972,#22973);
#19259=AXIS2_PLACEMENT_3D('',#49081,#22974,#22975);
#19260=AXIS2_PLACEMENT_3D('',#49089,#22976,#22977);
#19261=AXIS2_PLACEMENT_3D('',#49090,#22978,#22979);
#19262=AXIS2_PLACEMENT_3D('',#49092,#22980,#22981);
#19263=AXIS2_PLACEMENT_3D('',#49093,#22982,#22983);
#19264=AXIS2_PLACEMENT_3D('',#49094,#22984,#22985);
#19265=AXIS2_PLACEMENT_3D('',#49095,#22986,#22987);
#19266=AXIS2_PLACEMENT_3D('',#49096,#22988,#22989);
#19267=AXIS2_PLACEMENT_3D('',#49097,#22990,#22991);
#19268=AXIS2_PLACEMENT_3D('',#49098,#22992,#22993);
#19269=AXIS2_PLACEMENT_3D('',#49099,#22994,#22995);
#19270=AXIS2_PLACEMENT_3D('',#49100,#22996,#22997);
#19271=AXIS2_PLACEMENT_3D('',#49102,#22998,#22999);
#19272=AXIS2_PLACEMENT_3D('',#49103,#23000,#23001);
#19273=AXIS2_PLACEMENT_3D('',#49104,#23002,#23003);
#19274=AXIS2_PLACEMENT_3D('',#49105,#23004,#23005);
#19275=AXIS2_PLACEMENT_3D('',#49106,#23006,#23007);
#19276=AXIS2_PLACEMENT_3D('',#49107,#23008,#23009);
#19277=AXIS2_PLACEMENT_3D('',#49108,#23010,#23011);
#19278=AXIS2_PLACEMENT_3D('',#49116,#23012,#23013);
#19279=AXIS2_PLACEMENT_3D('',#49117,#23014,#23015);
#19280=AXIS2_PLACEMENT_3D('',#49118,#23016,#23017);
#19281=AXIS2_PLACEMENT_3D('',#49119,#23018,#23019);
#19282=AXIS2_PLACEMENT_3D('',#49120,#23020,#23021);
#19283=AXIS2_PLACEMENT_3D('',#49121,#23022,#23023);
#19284=AXIS2_PLACEMENT_3D('',#49122,#23024,#23025);
#19285=AXIS2_PLACEMENT_3D('',#49123,#23026,#23027);
#19286=AXIS2_PLACEMENT_3D('',#49124,#23028,#23029);
#19287=AXIS2_PLACEMENT_3D('',#49125,#23030,#23031);
#19288=AXIS2_PLACEMENT_3D('',#49126,#23032,#23033);
#19289=AXIS2_PLACEMENT_3D('',#49127,#23034,#23035);
#19290=AXIS2_PLACEMENT_3D('',#49128,#23036,#23037);
#19291=AXIS2_PLACEMENT_3D('',#49129,#23038,#23039);
#19292=AXIS2_PLACEMENT_3D('',#49130,#23040,#23041);
#22825=DIRECTION('axis',(0.,0.,1.));
#22826=DIRECTION('refdir',(1.,0.,0.));
#22827=DIRECTION('center_axis',(1.24100495794237E-20,1.,9.9579925010296E-17));
#22828=DIRECTION('ref_axis',(-0.242093751695761,9.66207115918887E-17,-0.970252861572627));
#22829=DIRECTION('',(0.,-1.,0.));
#22830=DIRECTION('center_axis',(4.78776181462468E-8,-0.999999999999989,
1.38777575295897E-7));
#22831=DIRECTION('ref_axis',(0.228625617239181,-1.2415592080664E-7,-0.973514420613268));
#22832=DIRECTION('',(0.,1.,0.));
#22833=DIRECTION('center_axis',(4.78638686561428E-8,0.999999999999989,1.38744664442357E-7));
#22834=DIRECTION('ref_axis',(-0.657176856530054,1.36031932324909E-7,-0.753736412309541));
#22835=DIRECTION('center_axis',(-0.988756381047007,0.,0.149535343443703));
#22836=DIRECTION('ref_axis',(0.149535343443703,0.,0.988756381047007));
#22837=DIRECTION('',(-0.149535343443703,0.,-0.988756381047007));
#22838=DIRECTION('',(0.,-1.,0.));
#22839=DIRECTION('',(-0.149535343443703,0.,-0.988756381047007));
#22840=DIRECTION('',(0.,-1.,0.));
#22841=DIRECTION('center_axis',(-0.754320837054538,0.,0.656505959443889));
#22842=DIRECTION('ref_axis',(0.656505959443889,0.,0.754320837054538));
#22843=DIRECTION('',(0.,-1.,0.));
#22844=DIRECTION('',(-0.656505959443889,0.,-0.754320837054538));
#22845=DIRECTION('',(0.,-1.,0.));
#22846=DIRECTION('',(-0.656505959443889,0.,-0.754320837054538));
#22847=DIRECTION('center_axis',(0.,-1.,0.));
#22848=DIRECTION('ref_axis',(0.,0.,-1.));
#22849=DIRECTION('center_axis',(0.,-1.,0.));
#22850=DIRECTION('ref_axis',(0.,0.,-1.));
#22851=DIRECTION('',(0.,-1.,0.));
#22852=DIRECTION('center_axis',(0.,-1.,0.));
#22853=DIRECTION('ref_axis',(0.,0.,-1.));
#22854=DIRECTION('center_axis',(0.754320837054538,0.,0.656505959443889));
#22855=DIRECTION('ref_axis',(0.656505959443889,0.,-0.754320837054538));
#22856=DIRECTION('',(-0.656505959443889,0.,0.754320837054538));
#22857=DIRECTION('',(0.,-1.,0.));
#22858=DIRECTION('',(-0.656505959443889,0.,0.754320837054538));
#22859=DIRECTION('center_axis',(0.988756381047007,0.,0.149535343443703));
#22860=DIRECTION('ref_axis',(0.149535343443703,0.,-0.988756381047007));
#22861=DIRECTION('',(-0.149535343443703,0.,0.988756381047007));
#22862=DIRECTION('',(0.,-1.,0.));
#22863=DIRECTION('',(-0.149535343443703,0.,0.988756381047007));
#22864=DIRECTION('',(0.,-1.,0.));
#22865=DIRECTION('center_axis',(-1.24149291915094E-20,1.,9.9579925010296E-17));
#22866=DIRECTION('ref_axis',(0.242093751716637,9.66207127726939E-17,-0.970252861567418));
#22867=DIRECTION('',(0.,-1.,0.));
#22868=DIRECTION('center_axis',(-4.78638689058599E-8,-0.999999999999989,
1.38744669549957E-7));
#22869=DIRECTION('ref_axis',(0.657176856532881,-1.36031936363378E-7,-0.753736412307076));
#22870=DIRECTION('',(0.,1.,0.));
#22871=DIRECTION('center_axis',(-4.78776226059778E-8,0.999999999999989,
1.38777586767972E-7));
#22872=DIRECTION('ref_axis',(-0.228625617218267,1.24155931198126E-7,-0.97351442061818));
#22873=DIRECTION('center_axis',(0.,-1.,0.));
#22874=DIRECTION('ref_axis',(-4.27550288255207E-14,0.,1.));
#22875=DIRECTION('center_axis',(0.,-1.,0.));
#22876=DIRECTION('ref_axis',(0.,0.,-1.));
#22877=DIRECTION('center_axis',(0.,-1.,0.));
#22878=DIRECTION('ref_axis',(0.,0.,-1.));
#22879=DIRECTION('center_axis',(0.,-1.,0.));
#22880=DIRECTION('ref_axis',(0.,0.,-1.));
#22881=DIRECTION('center_axis',(0.,-1.,0.));
#22882=DIRECTION('ref_axis',(0.,0.,-1.));
#22883=DIRECTION('center_axis',(0.,-1.,0.));
#22884=DIRECTION('ref_axis',(-0.319023595909223,0.,-0.947746772747419));
#22885=DIRECTION('center_axis',(0.,-1.,0.));
#22886=DIRECTION('ref_axis',(-0.319023595909223,0.,-0.947746772747419));
#22887=DIRECTION('',(-0.149535343443703,0.,-0.988756381047007));
#22888=DIRECTION('',(-0.656505959443889,0.,-0.754320837054538));
#22889=DIRECTION('center_axis',(0.,-1.,0.));
#22890=DIRECTION('ref_axis',(0.,0.,-1.));
#22891=DIRECTION('',(-0.656505959443889,0.,0.754320837054538));
#22892=DIRECTION('',(-0.149535343443703,0.,0.988756381047007));
#22893=DIRECTION('center_axis',(0.,-1.,0.));
#22894=DIRECTION('ref_axis',(0.,0.,-1.));
#22895=DIRECTION('center_axis',(0.,-1.,0.));
#22896=DIRECTION('ref_axis',(0.,0.,-1.));
#22897=DIRECTION('',(-0.656505959443889,0.,-0.754320837054538));
#22898=DIRECTION('',(-0.149535343443703,0.,-0.988756381047007));
#22899=DIRECTION('center_axis',(0.,-1.,0.));
#22900=DIRECTION('ref_axis',(0.,0.,-1.));
#22901=DIRECTION('center_axis',(0.,1.,0.));
#22902=DIRECTION('ref_axis',(-0.319023595909249,0.,0.94774677274741));
#22903=DIRECTION('center_axis',(0.,1.,0.));
#22904=DIRECTION('ref_axis',(-0.319023595909249,0.,0.94774677274741));
#22905=DIRECTION('',(-0.149535343443703,0.,0.988756381047007));
#22906=DIRECTION('',(-0.656505959443889,0.,0.754320837054538));
#22907=DIRECTION('center_axis',(0.,-1.,0.));
#22908=DIRECTION('ref_axis',(0.,0.,-1.));
#22909=DIRECTION('center_axis',(0.,-1.,0.));
#22910=DIRECTION('ref_axis',(0.,0.,-1.));
#22911=DIRECTION('center_axis',(0.,1.,0.));
#22912=DIRECTION('ref_axis',(0.,0.,1.));
#22913=DIRECTION('center_axis',(0.,-1.,0.));
#22914=DIRECTION('ref_axis',(0.,0.,-1.));
#22915=DIRECTION('center_axis',(0.,-1.,0.));
#22916=DIRECTION('ref_axis',(0.,0.,-1.));
#22917=DIRECTION('',(0.,1.,0.));
#22918=DIRECTION('center_axis',(0.,-1.,0.));
#22919=DIRECTION('ref_axis',(0.,0.,-1.));
#22920=DIRECTION('center_axis',(0.,-1.,0.));
#22921=DIRECTION('ref_axis',(0.,0.,-1.));
#22922=DIRECTION('center_axis',(-0.149535343443703,0.,0.988756381047007));
#22923=DIRECTION('ref_axis',(0.988756381047007,0.,0.149535343443703));
#22924=DIRECTION('center_axis',(-0.149535343443704,0.,0.988756381047007));
#22925=DIRECTION('ref_axis',(0.988756381047007,0.,0.149535343443704));
#22926=DIRECTION('center_axis',(0.149535343443704,5.36005908195038E-16,
-0.988756381047007));
#22927=DIRECTION('ref_axis',(-0.988756381047007,1.21230624919584E-32,-0.149535343443704));
#22928=DIRECTION('center_axis',(0.577350269189623,0.577350269189631,0.577350269189624));
#22929=DIRECTION('ref_axis',(-0.707106781186548,0.,0.707106781186547));
#22930=DIRECTION('center_axis',(0.,1.,0.));
#22931=DIRECTION('ref_axis',(0.,0.,1.));
#22932=DIRECTION('center_axis',(0.,1.,0.));
#22933=DIRECTION('ref_axis',(0.,0.,1.));
#22934=DIRECTION('center_axis',(0.,1.,0.));
#22935=DIRECTION('ref_axis',(0.,0.,1.));
#22936=DIRECTION('center_axis',(-0.65650595944389,0.,0.754320837054537));
#22937=DIRECTION('ref_axis',(0.754320837054537,0.,0.656505959443889));
#22938=DIRECTION('center_axis',(0.,-1.,0.));
#22939=DIRECTION('ref_axis',(-0.693236209136321,0.,0.720710453887206));
#22940=DIRECTION('center_axis',(0.,-1.,0.));
#22941=DIRECTION('ref_axis',(0.,0.,-1.));
#22942=DIRECTION('center_axis',(0.,-1.,0.));
#22943=DIRECTION('ref_axis',(0.242097618474639,0.,-0.970251896740691));
#22944=DIRECTION('center_axis',(-0.656505959443889,0.,0.754320837054538));
#22945=DIRECTION('ref_axis',(0.754320837054538,0.,0.656505959443889));
#22946=DIRECTION('center_axis',(0.656505959443889,0.,-0.754320837054538));
#22947=DIRECTION('ref_axis',(-0.754320837054538,0.,-0.656505959443889));
#22948=DIRECTION('center_axis',(0.,-1.,0.));
#22949=DIRECTION('ref_axis',(0.,0.,-1.));
#22950=DIRECTION('center_axis',(0.,-1.,0.));
#22951=DIRECTION('ref_axis',(0.,0.,-1.));
#22952=DIRECTION('center_axis',(0.149535343443703,0.,-0.988756381047007));
#22953=DIRECTION('ref_axis',(-0.988756381047007,0.,-0.149535343443703));
#22954=DIRECTION('center_axis',(-0.149535343443704,-5.36005908195038E-15,
0.988756381047007));
#22955=DIRECTION('ref_axis',(0.988756381047007,-3.32168718654534E-32,0.149535343443704));
#22956=DIRECTION('center_axis',(0.149535343443707,0.,-0.988756381047006));
#22957=DIRECTION('ref_axis',(-0.988756381047006,0.,-0.149535343443707));
#22958=DIRECTION('center_axis',(0.577350269189625,0.577350269189626,0.577350269189626));
#22959=DIRECTION('ref_axis',(-0.707106781186548,0.,0.707106781186547));
#22960=DIRECTION('center_axis',(0.,-1.,0.));
#22961=DIRECTION('ref_axis',(-7.27572790734007E-5,0.,0.999999997353189));
#22962=DIRECTION('center_axis',(-0.759157852463309,0.000273278785289962,
0.650906506621344));
#22963=DIRECTION('ref_axis',(0.011467416751576,0.999850324991952,0.012954766170509));
#22964=DIRECTION('center_axis',(0.,-1.,0.));
#22965=DIRECTION('ref_axis',(0.,0.,-1.));
#22966=DIRECTION('center_axis',(0.656505959443889,0.,0.754320837054538));
#22967=DIRECTION('ref_axis',(0.754320837054538,0.,-0.656505959443889));
#22968=DIRECTION('center_axis',(0.,-1.,4.33680868994202E-15));
#22969=DIRECTION('ref_axis',(0.,-4.33680868994202E-15,-1.));
#22970=DIRECTION('center_axis',(-0.656505959443889,2.86242701599967E-15,
0.754320837054538));
#22971=DIRECTION('ref_axis',(0.754320837054538,8.45944254531623E-32,0.656505959443889));
#22972=DIRECTION('center_axis',(1.43818211772392E-17,-1.,-2.7292332891214E-17));
#22973=DIRECTION('ref_axis',(0.242098473658204,2.63898515742187E-17,-0.970251683354565));
#22974=DIRECTION('center_axis',(8.39371644022886E-16,-1.,-2.61255151017137E-16));
#22975=DIRECTION('ref_axis',(-0.24209847365972,0.,-0.970251683354187));
#22976=DIRECTION('center_axis',(-0.149535343443703,0.,-0.988756381047007));
#22977=DIRECTION('ref_axis',(-0.988756381047007,0.,0.149535343443703));
#22978=DIRECTION('center_axis',(-0.149535343443694,0.,-0.988756381047008));
#22979=DIRECTION('ref_axis',(-0.988756381047008,0.,0.149535343443694));
#22980=DIRECTION('center_axis',(0.149535343443704,6.00856525885051E-15,
0.988756381047007));
#22981=DIRECTION('ref_axis',(0.988756381047007,-1.58953417427367E-31,-0.149535343443704));
#22982=DIRECTION('center_axis',(0.149535343443704,6.00856525885051E-15,
0.988756381047007));
#22983=DIRECTION('ref_axis',(0.988756381047007,-1.58953417427367E-31,-0.149535343443704));
#22984=DIRECTION('center_axis',(-0.656505959443889,0.,-0.754320837054538));
#22985=DIRECTION('ref_axis',(-0.754320837054538,0.,0.656505959443889));
#22986=DIRECTION('center_axis',(0.656505959443889,1.06165855076284E-14,
0.754320837054538));
#22987=DIRECTION('ref_axis',(0.754320837054538,-1.58155227462586E-31,-0.656505959443889));
#22988=DIRECTION('center_axis',(0.656505959443889,0.,-0.754320837054538));
#22989=DIRECTION('ref_axis',(-0.754320837054538,0.,-0.656505959443889));
#22990=DIRECTION('center_axis',(0.656505959443889,0.,-0.754320837054538));
#22991=DIRECTION('ref_axis',(-0.754320837054538,0.,-0.656505959443889));
#22992=DIRECTION('center_axis',(0.,-1.,0.));
#22993=DIRECTION('ref_axis',(-7.273230047561E-5,0.,0.999999997355006));
#22994=DIRECTION('center_axis',(-0.759157804384072,-0.000273319894445015,
0.650906562679307));
#22995=DIRECTION('ref_axis',(0.650906589214572,-1.08983609746617E-5,0.759157830756081));
#22996=DIRECTION('center_axis',(0.577350269189623,0.577350269189631,0.577350269189624));
#22997=DIRECTION('ref_axis',(-0.707106781186548,0.,0.707106781186547));
#22998=DIRECTION('center_axis',(-0.408248290463864,0.816496580927726,-0.408248290463862));
#22999=DIRECTION('ref_axis',(0.707106781186546,0.,-0.707106781186549));
#23000=DIRECTION('center_axis',(0.,1.,0.));
#23001=DIRECTION('ref_axis',(0.,0.,1.));
#23002=DIRECTION('center_axis',(-4.33680868994204E-15,1.,-8.67361737988409E-15));
#23003=DIRECTION('ref_axis',(0.,1.73472347597681E-14,1.));
#23004=DIRECTION('center_axis',(0.,1.,0.));
#23005=DIRECTION('ref_axis',(0.,0.,1.));
#23006=DIRECTION('center_axis',(0.,-1.,0.));
#23007=DIRECTION('ref_axis',(0.,0.,-1.));
#23008=DIRECTION('center_axis',(0.656505959443889,0.,0.754320837054538));
#23009=DIRECTION('ref_axis',(0.754320837054538,0.,-0.656505959443889));
#23010=DIRECTION('center_axis',(0.,-1.,0.));
#23011=DIRECTION('ref_axis',(-0.242097618470637,0.,-0.970251896741689));
#23012=DIRECTION('center_axis',(0.,-1.,0.));
#23013=DIRECTION('ref_axis',(0.693236209130818,0.,0.720710453892499));
#23014=DIRECTION('center_axis',(0.,-1.,0.));
#23015=DIRECTION('ref_axis',(0.,0.,-1.));
#23016=DIRECTION('center_axis',(0.,-1.,0.));
#23017=DIRECTION('ref_axis',(0.,0.,-1.));
#23018=DIRECTION('center_axis',(0.,-1.,0.));
#23019=DIRECTION('ref_axis',(0.,0.,-1.));
#23020=DIRECTION('center_axis',(0.656505959443889,0.,0.754320837054538));
#23021=DIRECTION('ref_axis',(0.754320837054538,0.,-0.656505959443889));
#23022=DIRECTION('center_axis',(0.656505959443887,0.,0.75432083705454));
#23023=DIRECTION('ref_axis',(0.75432083705454,0.,-0.656505959443887));
#23024=DIRECTION('center_axis',(0.577350269189625,0.577350269189626,0.577350269189626));
#23025=DIRECTION('ref_axis',(-0.707106781186548,0.,0.707106781186547));
#23026=DIRECTION('center_axis',(0.1495353434437,0.,0.988756381047007));
#23027=DIRECTION('ref_axis',(0.988756381047007,0.,-0.1495353434437));
#23028=DIRECTION('center_axis',(0.,-1.,-3.25260651745651E-15));
#23029=DIRECTION('ref_axis',(0.,3.25260651745651E-15,-1.));
#23030=DIRECTION('center_axis',(-0.149535343443704,2.68002954097519E-15,
-0.988756381047007));
#23031=DIRECTION('ref_axis',(-0.988756381047007,-1.66084359327267E-32,0.149535343443704));
#23032=DIRECTION('center_axis',(0.149535343443703,0.,0.988756381047007));
#23033=DIRECTION('ref_axis',(0.988756381047007,0.,-0.149535343443703));
#23034=DIRECTION('center_axis',(0.,-1.,0.));
#23035=DIRECTION('ref_axis',(0.,0.,-1.));
#23036=DIRECTION('center_axis',(-1.,0.,-1.22464679914735E-16));
#23037=DIRECTION('ref_axis',(-1.22464679914735E-16,0.,1.));
#23038=DIRECTION('center_axis',(0.,-1.,0.));
#23039=DIRECTION('ref_axis',(0.,0.,-1.));
#23040=DIRECTION('center_axis',(-1.,0.,-1.22464679914735E-16));
#23041=DIRECTION('ref_axis',(-1.22464679914735E-16,0.,1.));
#48886=CARTESIAN_POINT('',(0.,0.,0.));
#48887=CARTESIAN_POINT('Origin',(0.0026795695442083,0.0119999999976374,
0.00311832636829977));
#48888=CARTESIAN_POINT('',(0.0011104902728708,0.0118999999786958,0.00129548235688735));
#48889=CARTESIAN_POINT('',(0.0011104897024608,0.000100000021359172,0.00129548157965629));
#48890=CARTESIAN_POINT('',(0.00111150801408478,0.0119,0.00129670923842467));
#48891=CARTESIAN_POINT('',(0.00320791856642742,0.000100000046696322,0.000774301462227049));
#48892=CARTESIAN_POINT('Origin',(0.00266641386133884,0.000100000326685605,
0.00308004099065544));
#48893=CARTESIAN_POINT('',(0.00320786705247145,0.0118999999521473,0.000774537053797754));
#48894=CARTESIAN_POINT('',(0.00320887657816064,0.0001,0.000769953068500355));
#48895=CARTESIAN_POINT('Origin',(0.00266641994550595,0.0118999996733985,
0.00308005675377107));
#48896=CARTESIAN_POINT('Origin',(0.00334795260328877,0.012,0.000799258762279974));
#48897=CARTESIAN_POINT('',(0.00332640074788228,0.0001,0.000656753759343362));
#48898=CARTESIAN_POINT('',(0.00317081887252197,0.0001,-0.000371983450837843));
#48899=CARTESIAN_POINT('',(0.00316646966616483,0.0001,-0.000400741237720026));
#48900=CARTESIAN_POINT('',(0.00317081887252197,0.0119,-0.000371983450837843));
#48901=CARTESIAN_POINT('',(0.00317081887252197,0.012,-0.000371983450837842));
#48902=CARTESIAN_POINT('',(0.00332640074788228,0.0119,0.000656753759343362));
#48903=CARTESIAN_POINT('',(0.00334795260328877,0.0119,0.000799258762279974));
#48904=CARTESIAN_POINT('',(0.00332640074788228,0.012,0.000656753759343362));
#48905=CARTESIAN_POINT('Origin',(0.00200017452605719,0.012,-0.00174080634098864));
#48906=CARTESIAN_POINT('',(0.00314737531812273,0.0119,-0.000422680512437861));
#48907=CARTESIAN_POINT('',(0.00314737531812273,0.0001,-0.000422680512437861));
#48908=CARTESIAN_POINT('',(0.00314737531812273,0.012,-0.000422680512437861));
#48909=CARTESIAN_POINT('',(0.00200017452605719,0.0001,-0.00174080634098864));
#48910=CARTESIAN_POINT('',(0.00200017452605719,0.0001,-0.00174080634098864));
#48911=CARTESIAN_POINT('',(0.00200017452605719,0.0119,-0.00174080634098864));
#48912=CARTESIAN_POINT('',(0.00200017452605719,0.012,-0.00174080634098864));
#48913=CARTESIAN_POINT('',(0.00200017452605719,0.0119,-0.00174080634098864));
#48914=CARTESIAN_POINT('Origin',(0.,0.012,0.));
#48915=CARTESIAN_POINT('',(-0.00200017452605719,0.0001,-0.00174080634098864));
#48916=CARTESIAN_POINT('Origin',(0.,0.0001,0.));
#48917=CARTESIAN_POINT('',(-0.00200017452605719,0.0119,-0.00174080634098864));
#48918=CARTESIAN_POINT('',(-0.00200017452605719,0.012,-0.00174080634098864));
#48919=CARTESIAN_POINT('Origin',(0.,0.0119,0.));
#48920=CARTESIAN_POINT('Origin',(-0.00200017452605719,0.012,-0.00174080634098864));
#48921=CARTESIAN_POINT('',(-0.00314737531812273,0.0001,-0.000422680512437861));
#48922=CARTESIAN_POINT('',(-0.00316646966616483,0.0001,-0.000400741237720025));
#48923=CARTESIAN_POINT('',(-0.00314737531812273,0.0119,-0.000422680512437861));
#48924=CARTESIAN_POINT('',(-0.00314737531812273,0.012,-0.000422680512437861));
#48925=CARTESIAN_POINT('',(-0.00200017452605719,0.0119,-0.00174080634098864));
#48926=CARTESIAN_POINT('Origin',(-0.00334795260328877,0.012,0.000799258762279975));
#48927=CARTESIAN_POINT('',(-0.00332640074788227,0.0119,0.000656753759343363));
#48928=CARTESIAN_POINT('',(-0.00317081887252197,0.0119,-0.000371983450837842));
#48929=CARTESIAN_POINT('',(-0.00334795260328877,0.0119,0.000799258762279975));
#48930=CARTESIAN_POINT('',(-0.00317081887252197,0.0001,-0.000371983450837842));
#48931=CARTESIAN_POINT('',(-0.00317081887252197,0.012,-0.000371983450837842));
#48932=CARTESIAN_POINT('',(-0.00332640074788227,0.0001,0.000656753759343363));
#48933=CARTESIAN_POINT('',(-0.00334795260328877,0.0001,0.000799258762279975));
#48934=CARTESIAN_POINT('',(-0.00332640074788227,0.012,0.000656753759343363));
#48935=CARTESIAN_POINT('Origin',(-0.00267956954438675,0.0119999999976374,
0.00311832636876968));
#48936=CARTESIAN_POINT('',(-0.00320791856642536,0.0118999999533037,0.000774301462240489));
#48937=CARTESIAN_POINT('',(-0.00320791920421998,0.000100000046677651,0.000774298724656522));
#48938=CARTESIAN_POINT('',(-0.00320887657816269,0.0119,0.000769953068500743));
#48939=CARTESIAN_POINT('',(-0.00111049188113299,0.000100000455445466,0.00129548100148887));
#48940=CARTESIAN_POINT('Origin',(-0.00266641994549533,0.000100000326601476,
0.0030800567537451));
#48941=CARTESIAN_POINT('',(-0.00111049131362328,0.0118999995438595,0.0012954802219009));
#48942=CARTESIAN_POINT('',(-0.00111150801408489,0.0001,0.00129670923842458));
#48943=CARTESIAN_POINT('Origin',(-0.00266641386137086,0.0118999996733144,
0.00308004099074208));
#48944=CARTESIAN_POINT('Origin',(0.,0.012,0.));
#48945=CARTESIAN_POINT('Origin',(0.,0.0001,0.));
#48946=CARTESIAN_POINT('Origin',(0.,0.0119,0.));
#48947=CARTESIAN_POINT('Origin',(0.00213706124849222,0.012,0.000772521431045073));
#48948=CARTESIAN_POINT('',(-0.00322752330024893,0.0119998704155119,0.000671715368343072));
#48949=CARTESIAN_POINT('',(-0.00308038924536576,0.0120000000376982,0.000647274389139154));
#48950=CARTESIAN_POINT('Ctrl Pts',(-0.00322752354088739,0.0119998703308515,
0.000671713719076399));
#48951=CARTESIAN_POINT('Ctrl Pts',(-0.00317812331295772,0.0119999770854659,
0.000662354121866401));
#48952=CARTESIAN_POINT('Ctrl Pts',(-0.00312908474940071,0.0120000000376982,
0.000654218836705111));
#48953=CARTESIAN_POINT('Ctrl Pts',(-0.00308038924536576,0.0120000000376982,
0.000647274389139154));
#48954=CARTESIAN_POINT('',(-0.00104643070386136,0.0119999950205632,0.0012207818227995));
#48955=CARTESIAN_POINT('Ctrl Pts',(-0.00308038924536576,0.0120000000376982,
0.000647274389139154));
#48956=CARTESIAN_POINT('Ctrl Pts',(-0.00280336974579476,0.0120000000376982,
0.000607768742208423));
#48957=CARTESIAN_POINT('Ctrl Pts',(-0.00253662303677809,0.0119999551733919,
0.000605951286767472));
#48958=CARTESIAN_POINT('Ctrl Pts',(-0.00228179200572747,0.0119999881420702,
0.000644022735642257));
#48959=CARTESIAN_POINT('Ctrl Pts',(-0.00192078189626786,0.0120000348476307,
0.000697957210846894));
#48960=CARTESIAN_POINT('Ctrl Pts',(-0.00158393163555709,0.0119999540372077,
0.0008335151744178));
#48961=CARTESIAN_POINT('Ctrl Pts',(-0.00127112647954639,0.011999958801516,
0.00104811133060204));
#48962=CARTESIAN_POINT('Ctrl Pts',(-0.00119465884940102,0.0119999599661878,
0.0011005710141667));
#48963=CARTESIAN_POINT('Ctrl Pts',(-0.00111968086511865,0.0119999715654864,
0.00115799258041393));
#48964=CARTESIAN_POINT('Ctrl Pts',(-0.00104643062837067,0.0119999850616897,
0.00122078173615864));
#48965=CARTESIAN_POINT('',(0.00104643070371687,0.0119999950154752,0.00122078182263315));
#48966=CARTESIAN_POINT('Origin',(0.,0.012,0.));
#48967=CARTESIAN_POINT('',(0.00308076069387804,0.012,0.000647255039318342));
#48968=CARTESIAN_POINT('Origin',(0.024699859933188,0.012,0.0685450159411535));
#48969=CARTESIAN_POINT('',(0.00322751928435601,0.0119998716555966,0.000671736604513569));
#48970=CARTESIAN_POINT('Origin',(0.024699859933188,0.012,0.0685450159411535));
#48971=CARTESIAN_POINT('',(0.00307194323441727,0.012,-0.000357029916493473));
#48972=CARTESIAN_POINT('',(0.00321804722080344,0.012,0.000609037673341061));
#48973=CARTESIAN_POINT('',(0.00192474244235174,0.012,-0.00167515574504426));
#48974=CARTESIAN_POINT('',(0.00322838106972541,0.012,-0.00017728391848822));
#48975=CARTESIAN_POINT('',(-0.00192474244235174,0.012,-0.00167515574504426));
#48976=CARTESIAN_POINT('Origin',(0.,0.012,0.));
#48977=CARTESIAN_POINT('',(-0.00307194323441727,0.012,-0.000357029916493472));
#48978=CARTESIAN_POINT('',(-0.00138623395388341,0.012,-0.00229389829861756));
#48979=CARTESIAN_POINT('',(-0.00312247434152602,0.012,-2.29085412752433E-5));
#48980=CARTESIAN_POINT('',(-1.34711147906209E-19,0.012,0.0011));
#48981=CARTESIAN_POINT('Origin',(0.,0.012,0.));
#48982=CARTESIAN_POINT('Origin',(0.00213706124849222,0.,0.000772521431045073));
#48983=CARTESIAN_POINT('',(0.00192474244235174,0.,-0.00167515574504426));
#48984=CARTESIAN_POINT('',(0.00307194323441727,0.,-0.000357029916493473));
#48985=CARTESIAN_POINT('',(0.00309103758245938,0.,-0.000335090641775636));
#48986=CARTESIAN_POINT('',(0.00322752330024892,1.29584488918668E-7,0.000671715368343146));
#48987=CARTESIAN_POINT('',(0.00324907696518407,0.,0.000814212296624345));
#48988=CARTESIAN_POINT('',(0.00308038924492918,-3.76981371119633E-11,0.000647274389076851));
#48989=CARTESIAN_POINT('Ctrl Pts',(0.00322752354088737,1.29669149337175E-7,
0.000671713719076455));
#48990=CARTESIAN_POINT('Ctrl Pts',(0.00317812331281008,2.29145342387538E-8,
0.000662354121838435));
#48991=CARTESIAN_POINT('Ctrl Pts',(0.0031290847491076,-3.7698137119178E-11,
0.000654218836656452));
#48992=CARTESIAN_POINT('Ctrl Pts',(0.00308038924492918,-3.76981371195528E-11,
0.000647274389076851));
#48993=CARTESIAN_POINT('',(0.00104643062837068,1.49383102941193E-8,0.00122078173615864));
#48994=CARTESIAN_POINT('Ctrl Pts',(0.00308038924492918,-3.76981371195528E-11,
0.000647274389076851));
#48995=CARTESIAN_POINT('Ctrl Pts',(0.00280336974551912,-3.76981371216846E-11,
0.000607768742207853));
#48996=CARTESIAN_POINT('Ctrl Pts',(0.00253662303665133,4.48266081172561E-8,
0.000605951286787511));
#48997=CARTESIAN_POINT('Ctrl Pts',(0.00228179200573768,1.18579298942923E-8,
0.000644022735640731));
#48998=CARTESIAN_POINT('Ctrl Pts',(0.00192078189628118,-3.48476306147057E-8,
0.000697957210843341));
#48999=CARTESIAN_POINT('Ctrl Pts',(0.00158393163557307,4.59627924215703E-8,
0.000833515174410873));
#49000=CARTESIAN_POINT('Ctrl Pts',(0.00127112647956448,4.11984840427545E-8,
0.00104811133058969));
#49001=CARTESIAN_POINT('Ctrl Pts',(0.00119465884941284,4.00338121566248E-8,
0.00110057101415767));
#49002=CARTESIAN_POINT('Ctrl Pts',(0.00111968086512442,2.84345135863231E-8,
0.00115799258040899));
#49003=CARTESIAN_POINT('Ctrl Pts',(0.00104643062837068,1.49383102941041E-8,
0.00122078173615864));
#49004=CARTESIAN_POINT('',(-0.00104643079757785,0.,0.00122078193166094));
#49005=CARTESIAN_POINT('Origin',(0.,0.,0.));
#49006=CARTESIAN_POINT('',(-0.0030807606937324,0.,0.000647255039297434));
#49007=CARTESIAN_POINT('Origin',(-0.0246998599330348,0.,0.0685450159406926));
#49008=CARTESIAN_POINT('',(-0.00322751928435599,1.28344403638389E-7,0.00067173660451365));
#49009=CARTESIAN_POINT('Origin',(-0.0246998599330348,0.,0.0685450159406926));
#49010=CARTESIAN_POINT('',(-0.00307194323441727,0.,-0.000357029916493471));
#49011=CARTESIAN_POINT('',(-0.00306759402806013,0.,-0.000385787703375655));
#49012=CARTESIAN_POINT('',(-0.00192474244235174,0.,-0.00167515574504426));
#49013=CARTESIAN_POINT('',(-0.00192474244235174,0.,-0.00167515574504426));
#49014=CARTESIAN_POINT('Origin',(0.,0.,0.));
#49015=CARTESIAN_POINT('',(-1.34711147906209E-19,0.,0.0011));
#49016=CARTESIAN_POINT('Origin',(0.,0.,0.));
#49017=CARTESIAN_POINT('Origin',(0.,0.,0.));
#49018=CARTESIAN_POINT('',(0.,0.0001,-0.001));
#49019=CARTESIAN_POINT('',(-1.22464679914735E-19,0.0001,0.001));
#49020=CARTESIAN_POINT('Origin',(0.,0.0001,0.));
#49021=CARTESIAN_POINT('Origin',(0.,0.0001,0.));
#49022=CARTESIAN_POINT('',(0.,0.0119,-0.001));
#49023=CARTESIAN_POINT('',(-1.22464679914735E-19,0.,-0.001));
#49024=CARTESIAN_POINT('',(-1.22464679914735E-19,0.0119,0.001));
#49025=CARTESIAN_POINT('Origin',(0.,0.0119,0.));
#49026=CARTESIAN_POINT('Origin',(0.,0.0119,0.));
#49027=CARTESIAN_POINT('Origin',(-0.00312247434152602,0.0119,-2.29085412752431E-5));
#49028=CARTESIAN_POINT('Origin',(-0.00322752510977757,0.0119,0.000671707293687733));
#49029=CARTESIAN_POINT('Origin',(-0.00307194323441727,0.0119,-0.000357029916493472));
#49030=CARTESIAN_POINT('Origin',(-0.00322752510977757,0.0119,0.000671707293687733));
#49031=CARTESIAN_POINT('Ctrl Pts',(-0.00320773952081963,0.0118999999536822,
0.000775013487105381));
#49032=CARTESIAN_POINT('Ctrl Pts',(-0.00320773942939966,0.0119447930614053,
0.000775013876381884));
#49033=CARTESIAN_POINT('Ctrl Pts',(-0.00321413964601594,0.011986412579691,
0.000741829045057959));
#49034=CARTESIAN_POINT('Ctrl Pts',(-0.00322198939913603,0.0119969554905399,
0.000700795898891431));
#49035=CARTESIAN_POINT('Ctrl Pts',(-0.00322381747770655,0.0119994107613107,
0.00069123995311325));
#49036=CARTESIAN_POINT('Ctrl Pts',(-0.00322569246909101,0.0120003720874417,
0.000681395742799694));
#49037=CARTESIAN_POINT('Ctrl Pts',(-0.00322752330024893,0.0119998704155119,
0.000671715368343072));
#49038=CARTESIAN_POINT('Origin',(-0.00322752510977757,0.0119,0.000671707293687733));
#49039=CARTESIAN_POINT('Origin',(-0.00307194323441727,0.0119,-0.000357029916493472));
#49040=CARTESIAN_POINT('Origin',(-0.00307194323441727,0.0119,-0.000357029916493472));
#49041=CARTESIAN_POINT('Origin',(-0.00307194323441727,0.0119,-0.000357029916493472));
#49042=CARTESIAN_POINT('Origin',(-0.00322752510977757,0.006,0.000671707293687733));
#49043=CARTESIAN_POINT('Origin',(-0.00322752510977757,0.0001,0.000671707293687733));
#49044=CARTESIAN_POINT('Origin',(-0.00266641386136991,0.0119000008463731,
0.00308004099073934));
#49045=CARTESIAN_POINT('Ctrl Pts',(-0.00111150052572481,0.0119000008612573,
0.0012967156572246));
#49046=CARTESIAN_POINT('Ctrl Pts',(-0.00111167480720489,0.0119448666404984,
0.00129656576013425));
#49047=CARTESIAN_POINT('Ctrl Pts',(-0.00108952702596546,0.0119871861227217,
0.00127080632163187));
#49048=CARTESIAN_POINT('Ctrl Pts',(-0.00106139371099157,0.0119973373095639,
0.00123814749532547));
#49049=CARTESIAN_POINT('Ctrl Pts',(-0.00105648554162436,0.0119991082968914,
0.00123244980022645));
#49050=CARTESIAN_POINT('Ctrl Pts',(-0.00105145244004021,0.0119999999999997,
0.00122660881996128));
#49051=CARTESIAN_POINT('Ctrl Pts',(-0.00104643079716415,0.012,0.00122078193201883));
#49052=CARTESIAN_POINT('Origin',(-0.00138623395388341,0.0119,-0.00229389829861756));
#49053=CARTESIAN_POINT('Origin',(-0.00192474244235174,0.0119,-0.00167515574504426));
#49054=CARTESIAN_POINT('Origin',(-0.00307194323441727,0.012,-0.000357029916493472));
#49055=CARTESIAN_POINT('Origin',(-0.00307194323441727,0.0001,-0.000357029916493472));
#49056=CARTESIAN_POINT('Origin',(-0.00324907696518407,0.0001,0.000814212296624346));
#49057=CARTESIAN_POINT('Origin',(-0.00322752510977757,0.0001,0.000671707293687733));
#49058=CARTESIAN_POINT('Origin',(-0.00307194323441727,0.0001,-0.000357029916493471));
#49059=CARTESIAN_POINT('Origin',(-0.00322752510977757,9.99999999999988E-5,
0.000671707293687733));
#49060=CARTESIAN_POINT('Ctrl Pts',(-0.00322751928435599,1.2834440363839E-7,
0.00067173660451365));
#49061=CARTESIAN_POINT('Ctrl Pts',(-0.00321965722956229,-2.01559019057911E-6,
0.000713306122590413));
#49062=CARTESIAN_POINT('Ctrl Pts',(-0.00321120798733041,2.68608144209912E-5,
0.000756802444556823));
#49063=CARTESIAN_POINT('Ctrl Pts',(-0.00320864134773808,6.92989875928505E-5,
0.000770261872992935));
#49064=CARTESIAN_POINT('Ctrl Pts',(-0.00320804412466433,7.91737889874055E-5,
0.000773393703907348));
#49065=CARTESIAN_POINT('Ctrl Pts',(-0.00320774016282151,8.95773685078349E-5,
0.000775010844451836));
#49066=CARTESIAN_POINT('Ctrl Pts',(-0.00320774018409717,0.000100000046301422,
0.00077501075385594));
#49067=CARTESIAN_POINT('Origin',(0.,0.0119,0.));
#49068=CARTESIAN_POINT('Origin',(0.00104528387395555,0.0118999989257993,
0.00121948624514362));
#49069=CARTESIAN_POINT('Origin',(0.,0.0119,0.));
#49070=CARTESIAN_POINT('Origin',(0.00192474244235174,0.0119,-0.00167515574504426));
#49071=CARTESIAN_POINT('Origin',(-0.00307194323441727,0.0001,-0.000357029916493472));
#49072=CARTESIAN_POINT('Origin',(-0.00307194323441727,0.0001,-0.000357029916493472));
#49073=CARTESIAN_POINT('Origin',(-0.00266641994549438,9.9999153442383E-5,
0.00308005675374236));
#49074=CARTESIAN_POINT('Ctrl Pts',(-0.00104643079716283,0.,0.00122078193201997));
#49075=CARTESIAN_POINT('Ctrl Pts',(-0.00107521420056969,1.64668732167874E-15,
0.0012541809493851));
#49076=CARTESIAN_POINT('Ctrl Pts',(-0.00110310833148252,3.31402733155764E-5,
0.00128656285040545));
#49077=CARTESIAN_POINT('Ctrl Pts',(-0.00110978851162454,7.67397954013635E-5,
0.00129457061122281));
#49078=CARTESIAN_POINT('Ctrl Pts',(-0.00111095398235606,8.43464715416405E-5,
0.00129596770092087));
#49079=CARTESIAN_POINT('Ctrl Pts',(-0.00111153092065892,9.21715553007715E-5,
0.00129668951490891));
#49080=CARTESIAN_POINT('Ctrl Pts',(-0.00111150052324074,9.9999138547178E-5,
0.00129671565935386));
#49081=CARTESIAN_POINT('Origin',(0.002666419945505,0.0119000008465576,0.00308005675376833));
#49082=CARTESIAN_POINT('Ctrl Pts',(0.00322751928435601,0.0119998716555966,
0.00067173660451357));
#49083=CARTESIAN_POINT('Ctrl Pts',(0.00321965722956182,0.0120020155901889,
0.000713306122592838));
#49084=CARTESIAN_POINT('Ctrl Pts',(0.00321120798733032,0.0119731391855723,
0.000756802444558106));
#49085=CARTESIAN_POINT('Ctrl Pts',(0.00320864134773872,0.011930701012399,
0.000770261872990747));
#49086=CARTESIAN_POINT('Ctrl Pts',(0.00320804412466531,0.0119208262110068,
0.000773393703903478));
#49087=CARTESIAN_POINT('Ctrl Pts',(0.00320774016282266,0.0119104226314893,
0.000775010844447059));
#49088=CARTESIAN_POINT('Ctrl Pts',(0.00320774018409833,0.0118999999536986,
0.000775010753851165));
#49089=CARTESIAN_POINT('Origin',(0.00321804722080344,0.0119,0.000609037673341061));
#49090=CARTESIAN_POINT('Origin',(0.00307194323441727,0.0119,-0.000357029916493473));
#49091=CARTESIAN_POINT('',(0.00331869935185679,0.0119386927171885,0.000657918485985577));
#49092=CARTESIAN_POINT('Origin',(0.00322752510977757,0.0119,0.000671707293687733));
#49093=CARTESIAN_POINT('Origin',(0.00322752510977757,0.0119,0.000671707293687733));
#49094=CARTESIAN_POINT('Origin',(0.00322838106972541,0.0119,-0.00017728391848822));
#49095=CARTESIAN_POINT('Origin',(0.00307194323441727,0.0119,-0.000357029916493473));
#49096=CARTESIAN_POINT('Origin',(-0.00192474244235174,0.0001,-0.00167515574504426));
#49097=CARTESIAN_POINT('Origin',(-0.00192474244235174,0.0001,-0.00167515574504426));
#49098=CARTESIAN_POINT('Origin',(0.,0.0001,0.));
#49099=CARTESIAN_POINT('Origin',(0.00104528444769579,0.000100001075468891,
0.00121948692081579));
#49100=CARTESIAN_POINT('Origin',(0.00322752510977757,0.0119,0.000671707293687733));
#49101=CARTESIAN_POINT('',(0.00328526013669653,0.011957735026919,0.000729442320606695));
#49102=CARTESIAN_POINT('Origin',(0.00322752510977757,0.0119,0.000671707293687733));
#49103=CARTESIAN_POINT('Origin',(0.00322752510977783,0.0119,0.000671707293687782));
#49104=CARTESIAN_POINT('Origin',(0.00307194323441727,0.0119,-0.000357029916493473));
#49105=CARTESIAN_POINT('Origin',(0.00307194323441727,0.0119,-0.000357029916493473));
#49106=CARTESIAN_POINT('Origin',(0.,0.0001,0.));
#49107=CARTESIAN_POINT('Origin',(0.00192474244235174,0.0001,-0.00167515574504426));
#49108=CARTESIAN_POINT('Origin',(0.00266641386133789,9.99991536269668E-5,
0.0030800409906527));
#49109=CARTESIAN_POINT('Ctrl Pts',(0.00320773952081613,0.000100000046317807,
0.000775013487119797));
#49110=CARTESIAN_POINT('Ctrl Pts',(0.00320773942939615,5.52069385949101E-5,
0.000775013876396265));
#49111=CARTESIAN_POINT('Ctrl Pts',(0.00321413964601276,1.35874203120974E-5,
0.000741829045073119));
#49112=CARTESIAN_POINT('Ctrl Pts',(0.00322198939913204,3.04450946169635E-6,
0.00070079589891201));
#49113=CARTESIAN_POINT('Ctrl Pts',(0.00322381747770392,5.89238688465402E-7,
0.000691239953126957));
#49114=CARTESIAN_POINT('Ctrl Pts',(0.00322569246908978,-3.72087442654418E-7,
0.000681395742806229));
#49115=CARTESIAN_POINT('Ctrl Pts',(0.00322752330024892,1.29584488918648E-7,
0.000671715368343146));
#49116=CARTESIAN_POINT('Origin',(0.00322752510977757,0.006,0.000671707293687733));
#49117=CARTESIAN_POINT('Origin',(0.00322752510977757,0.0001,0.000671707293687733));
#49118=CARTESIAN_POINT('Origin',(0.00307194323441727,0.012,-0.000357029916493473));
#49119=CARTESIAN_POINT('Origin',(0.00307194323441727,0.0001,-0.000357029916493473));
#49120=CARTESIAN_POINT('Origin',(0.00192474244235174,0.0001,-0.00167515574504426));
#49121=CARTESIAN_POINT('Origin',(0.00307194323441727,0.0001,-0.000357029916493473));
#49122=CARTESIAN_POINT('Origin',(0.00322752510977757,9.99999999999988E-5,
0.000671707293687733));
#49123=CARTESIAN_POINT('Origin',(0.00322752510977757,0.0001,0.000671707293687732));
#49124=CARTESIAN_POINT('Origin',(0.00307194323441727,0.0001,-0.000357029916493473));
#49125=CARTESIAN_POINT('Origin',(0.00307194323441727,0.0001,-0.000357029916493473));
#49126=CARTESIAN_POINT('Origin',(0.00324907696518407,0.0001,0.000814212296624345));
#49127=CARTESIAN_POINT('Origin',(0.,0.0001,0.));
#49128=CARTESIAN_POINT('Origin',(-1.34711147906209E-19,0.0001,0.0011));
#49129=CARTESIAN_POINT('Origin',(0.,0.0119,0.));
#49130=CARTESIAN_POINT('Origin',(-1.34711147906209E-19,0.0119,0.0011));
#54561=UNCERTAINTY_MEASURE_WITH_UNIT(LENGTH_MEASURE(1.E-5),#54581,
'DISTANCE_ACCURACY_VALUE',
'Maximum model space distance between geometric entities at asserted c
onnectivities');
#54564=UNCERTAINTY_MEASURE_WITH_UNIT(LENGTH_MEASURE(1.E-5),#54581,
'DISTANCE_ACCURACY_VALUE',
'Maximum model space distance between geometric entities at asserted c
onnectivities');
#54577=(
GEOMETRIC_REPRESENTATION_CONTEXT(3)
GLOBAL_UNCERTAINTY_ASSIGNED_CONTEXT((#54561))
GLOBAL_UNIT_ASSIGNED_CONTEXT((#54581,#54582,#54583))
REPRESENTATION_CONTEXT('','3D')
);
#54580=(
GEOMETRIC_REPRESENTATION_CONTEXT(3)
GLOBAL_UNCERTAINTY_ASSIGNED_CONTEXT((#54564))
GLOBAL_UNIT_ASSIGNED_CONTEXT((#54581,#54582,#54583))
REPRESENTATION_CONTEXT('','3D')
);
#54581=(
LENGTH_UNIT()
NAMED_UNIT(*)
SI_UNIT($,.METRE.)
);
#54582=(
NAMED_UNIT(*)
PLANE_ANGLE_UNIT()
SI_UNIT($,.RADIAN.)
);
#54583=(
NAMED_UNIT(*)
SI_UNIT($,.STERADIAN.)
SOLID_ANGLE_UNIT()
);
#54596=SHAPE_DEFINITION_REPRESENTATION(#54611,#54641);
#54611=PRODUCT_DEFINITION_SHAPE('',$,#54657);
#54641=SHAPE_REPRESENTATION('',(#19199),#54577);
#54644=PRODUCT_DEFINITION_CONTEXT('part definition',#54691,'design');
#54657=PRODUCT_DEFINITION('Part_2','Part_2',#54672,#54644);
#54672=PRODUCT_DEFINITION_FORMATION('',$,#54705);
#54691=APPLICATION_CONTEXT(
'Core Data for Automotive Mechanical Design Process');
#54692=PRODUCT_CONTEXT('part definition',#54691,'mechanical');
#54705=PRODUCT('Part_2','Part_2','Part 2',(#54692));
#54712=PRESENTATION_STYLE_ASSIGNMENT((#54722));
#54722=SURFACE_STYLE_USAGE(.BOTH.,#54732);
#54732=SURFACE_SIDE_STYLE('',(#54742));
#54742=SURFACE_STYLE_FILL_AREA(#54752);
#54752=FILL_AREA_STYLE('Opaque(26,26,26)',(#54762));
#54762=FILL_AREA_STYLE_COLOUR('Opaque(26,26,26)',#54772);
#54772=COLOUR_RGB('Opaque(26,26,26)', 0.66274510, 0.83137255, 0.94901961);
ENDSEC;
END-ISO-10303-21;
